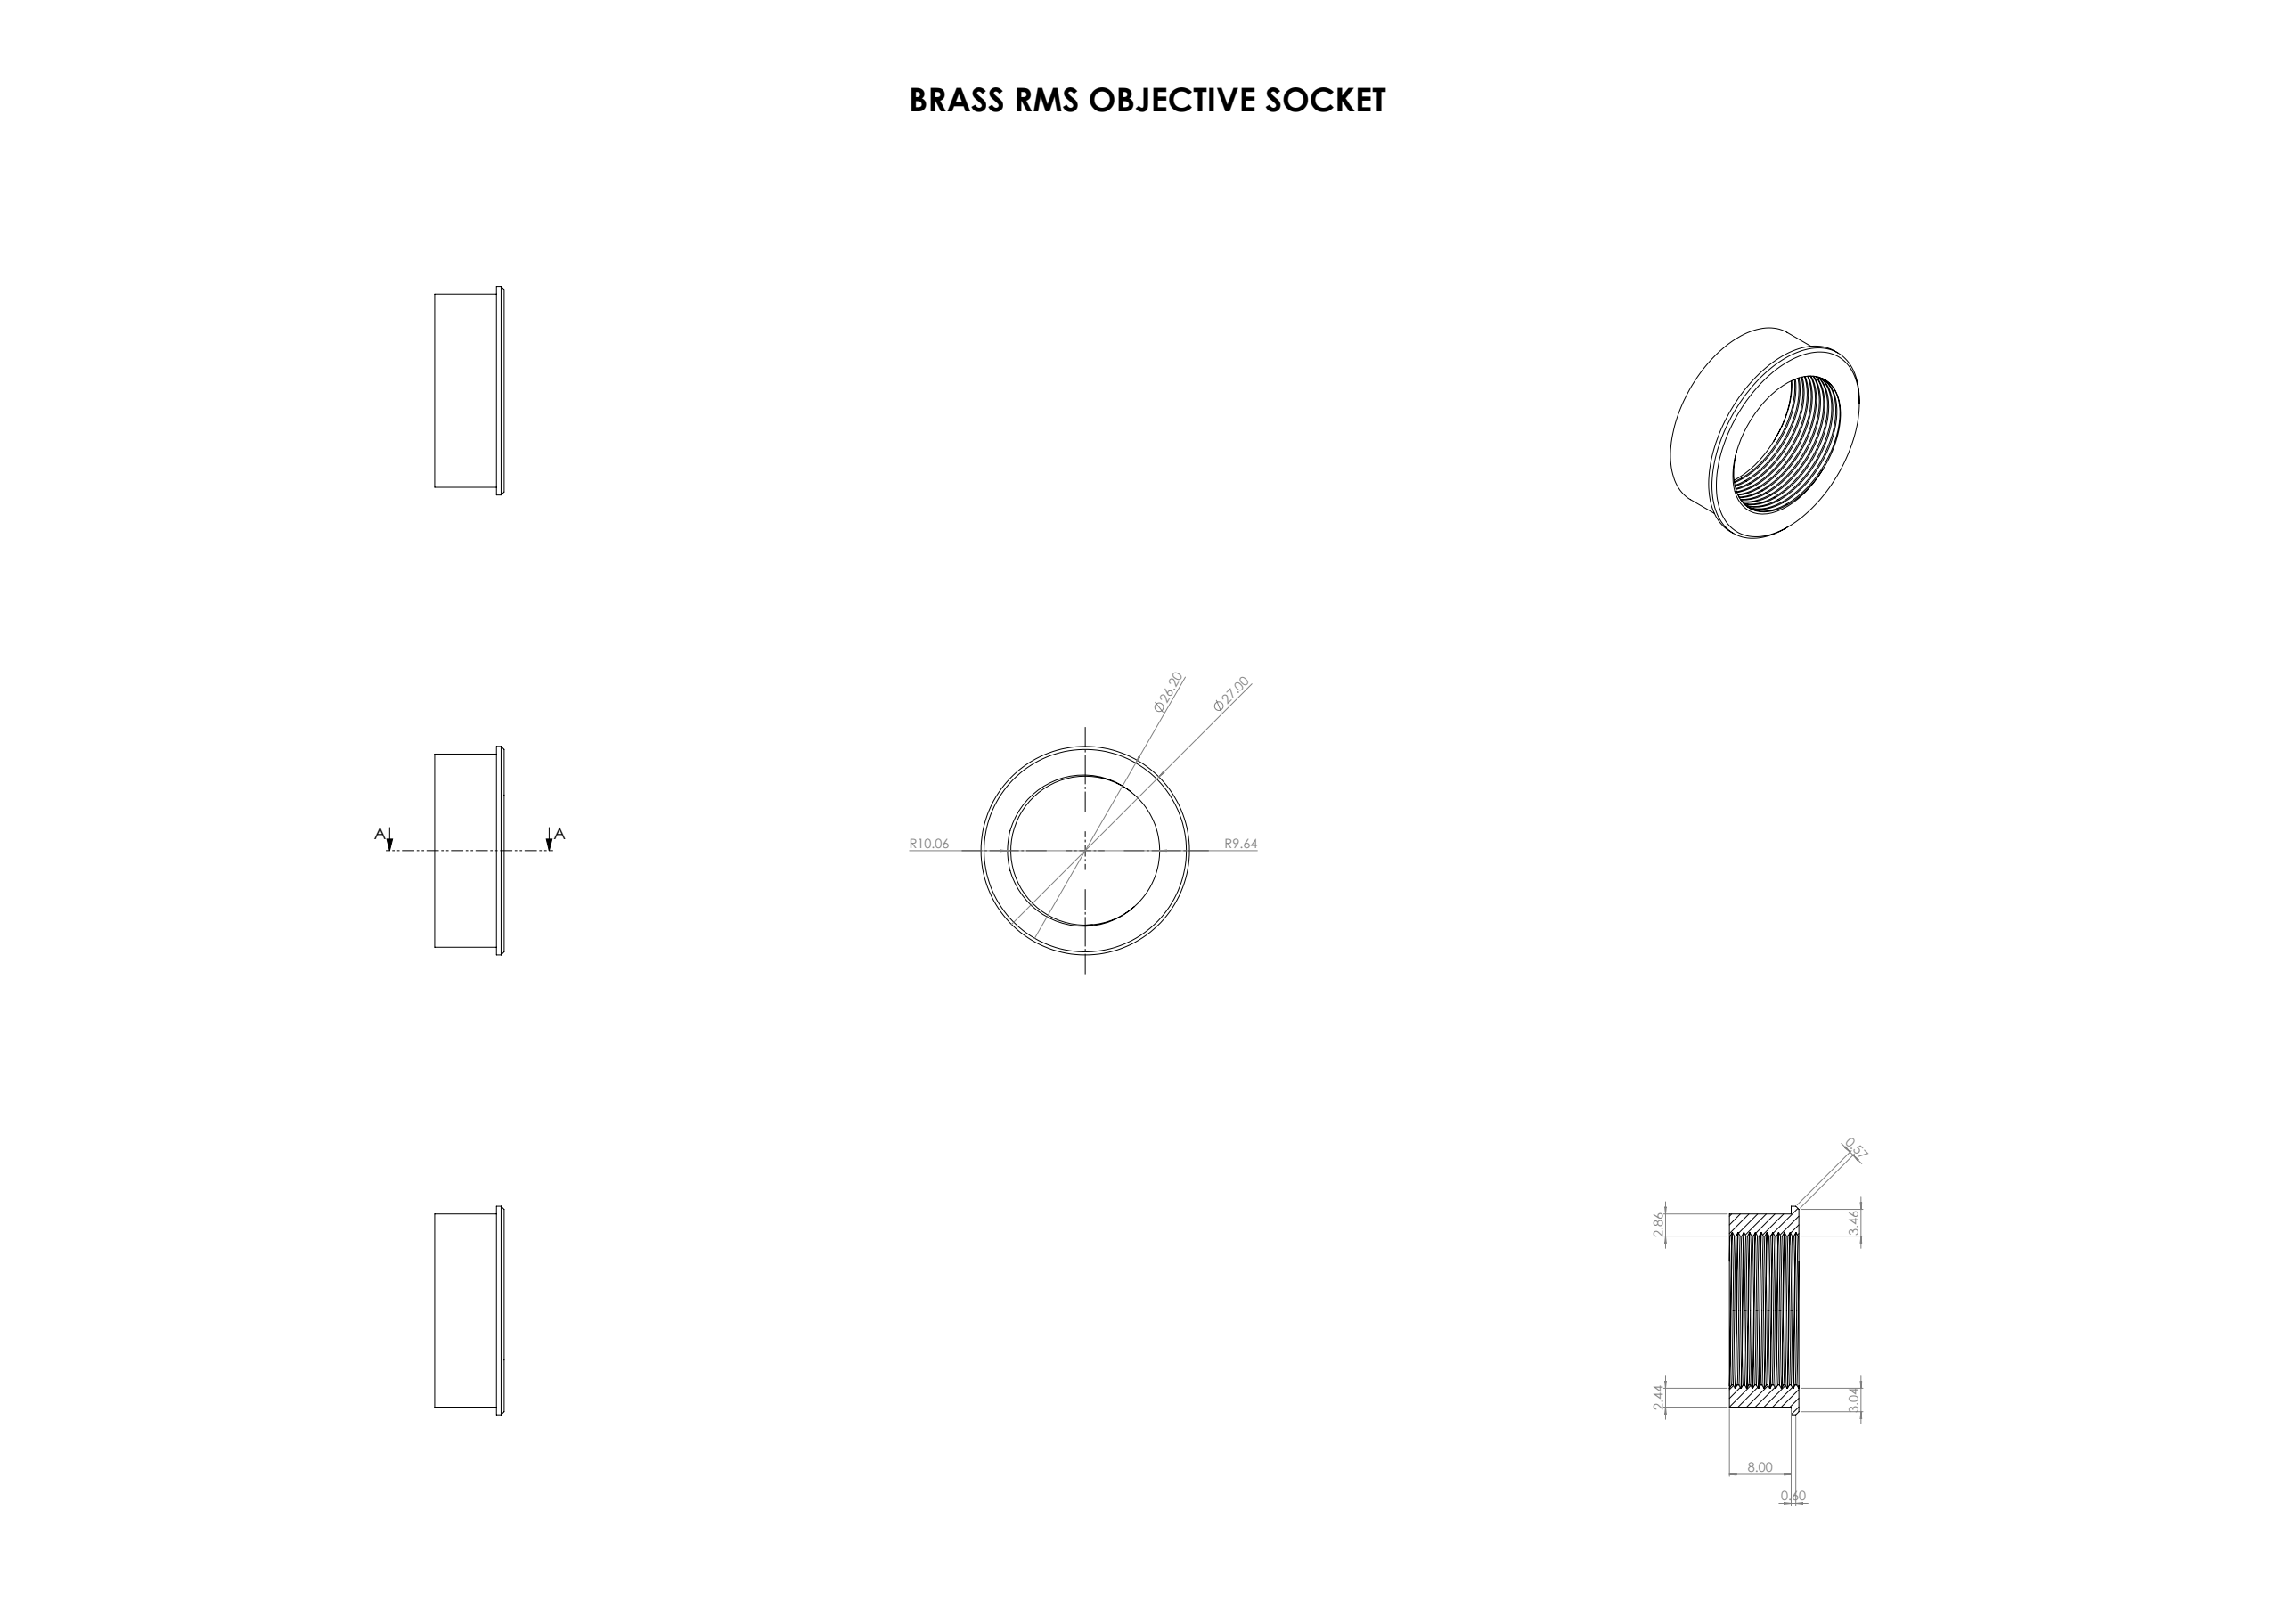
ISO-10303-21;
HEADER;
/* Generated by software containing ST-Developer
 * from STEP Tools, Inc. (www.steptools.com) 
 */

FILE_DESCRIPTION(
/* description */ (''),
/* implementation_level */ '2;1');

FILE_NAME(
/* name */ '03_Brass_RMS_Objective_Socket.step',
/* time_stamp */ '2026-10-21T02:03:06-07:00',
/* author */ (''),
/* organization */ (''),
/* preprocessor_version */ 'ST-DEVELOPER v20.2',
/* originating_system */ 'Autodesk Translation Framework v15.15.0.0',
/* authorisation */ '');

FILE_SCHEMA (('AUTOMOTIVE_DESIGN { 1 0 10303 214 3 1 1 }'));
ENDSEC;

DATA;
#10=MECHANICAL_DESIGN_GEOMETRIC_PRESENTATION_REPRESENTATION('',(#117),#38528);
#76=B_SPLINE_SURFACE_WITH_KNOTS('',3,3,((#30041,#30042,#30043,#30044,#30045,
#30046,#30047,#30048,#30049,#30050,#30051,#30052,#30053,#30054,#30055,#30056,
#30057,#30058,#30059,#30060,#30061,#30062,#30063,#30064,#30065,#30066,#30067,
#30068,#30069,#30070,#30071,#30072,#30073,#30074,#30075,#30076,#30077,#30078,
#30079,#30080,#30081,#30082,#30083,#30084,#30085,#30086,#30087,#30088,#30089,
#30090,#30091,#30092,#30093,#30094,#30095,#30096,#30097,#30098,#30099,#30100,
#30101,#30102,#30103,#30104,#30105,#30106,#30107,#30108,#30109,#30110,#30111,
#30112,#30113,#30114,#30115,#30116,#30117,#30118,#30119,#30120,#30121,#30122,
#30123,#30124,#30125,#30126,#30127,#30128,#30129,#30130,#30131,#30132,#30133,
#30134,#30135,#30136,#30137,#30138,#30139,#30140,#30141,#30142,#30143,#30144,
#30145,#30146,#30147,#30148,#30149,#30150,#30151,#30152,#30153,#30154,#30155,
#30156,#30157,#30158,#30159,#30160,#30161,#30162,#30163,#30164,#30165,#30166,
#30167,#30168,#30169,#30170,#30171,#30172,#30173,#30174,#30175,#30176,#30177,
#30178,#30179,#30180,#30181,#30182,#30183,#30184,#30185,#30186,#30187,#30188,
#30189,#30190,#30191,#30192,#30193,#30194,#30195,#30196,#30197,#30198,#30199),
(#30200,#30201,#30202,#30203,#30204,#30205,#30206,#30207,#30208,#30209,
#30210,#30211,#30212,#30213,#30214,#30215,#30216,#30217,#30218,#30219,#30220,
#30221,#30222,#30223,#30224,#30225,#30226,#30227,#30228,#30229,#30230,#30231,
#30232,#30233,#30234,#30235,#30236,#30237,#30238,#30239,#30240,#30241,#30242,
#30243,#30244,#30245,#30246,#30247,#30248,#30249,#30250,#30251,#30252,#30253,
#30254,#30255,#30256,#30257,#30258,#30259,#30260,#30261,#30262,#30263,#30264,
#30265,#30266,#30267,#30268,#30269,#30270,#30271,#30272,#30273,#30274,#30275,
#30276,#30277,#30278,#30279,#30280,#30281,#30282,#30283,#30284,#30285,#30286,
#30287,#30288,#30289,#30290,#30291,#30292,#30293,#30294,#30295,#30296,#30297,
#30298,#30299,#30300,#30301,#30302,#30303,#30304,#30305,#30306,#30307,#30308,
#30309,#30310,#30311,#30312,#30313,#30314,#30315,#30316,#30317,#30318,#30319,
#30320,#30321,#30322,#30323,#30324,#30325,#30326,#30327,#30328,#30329,#30330,
#30331,#30332,#30333,#30334,#30335,#30336,#30337,#30338,#30339,#30340,#30341,
#30342,#30343,#30344,#30345,#30346,#30347,#30348,#30349,#30350,#30351,#30352,
#30353,#30354,#30355,#30356,#30357,#30358),(#30359,#30360,#30361,#30362,
#30363,#30364,#30365,#30366,#30367,#30368,#30369,#30370,#30371,#30372,#30373,
#30374,#30375,#30376,#30377,#30378,#30379,#30380,#30381,#30382,#30383,#30384,
#30385,#30386,#30387,#30388,#30389,#30390,#30391,#30392,#30393,#30394,#30395,
#30396,#30397,#30398,#30399,#30400,#30401,#30402,#30403,#30404,#30405,#30406,
#30407,#30408,#30409,#30410,#30411,#30412,#30413,#30414,#30415,#30416,#30417,
#30418,#30419,#30420,#30421,#30422,#30423,#30424,#30425,#30426,#30427,#30428,
#30429,#30430,#30431,#30432,#30433,#30434,#30435,#30436,#30437,#30438,#30439,
#30440,#30441,#30442,#30443,#30444,#30445,#30446,#30447,#30448,#30449,#30450,
#30451,#30452,#30453,#30454,#30455,#30456,#30457,#30458,#30459,#30460,#30461,
#30462,#30463,#30464,#30465,#30466,#30467,#30468,#30469,#30470,#30471,#30472,
#30473,#30474,#30475,#30476,#30477,#30478,#30479,#30480,#30481,#30482,#30483,
#30484,#30485,#30486,#30487,#30488,#30489,#30490,#30491,#30492,#30493,#30494,
#30495,#30496,#30497,#30498,#30499,#30500,#30501,#30502,#30503,#30504,#30505,
#30506,#30507,#30508,#30509,#30510,#30511,#30512,#30513,#30514,#30515,#30516,
#30517),(#30518,#30519,#30520,#30521,#30522,#30523,#30524,#30525,#30526,
#30527,#30528,#30529,#30530,#30531,#30532,#30533,#30534,#30535,#30536,#30537,
#30538,#30539,#30540,#30541,#30542,#30543,#30544,#30545,#30546,#30547,#30548,
#30549,#30550,#30551,#30552,#30553,#30554,#30555,#30556,#30557,#30558,#30559,
#30560,#30561,#30562,#30563,#30564,#30565,#30566,#30567,#30568,#30569,#30570,
#30571,#30572,#30573,#30574,#30575,#30576,#30577,#30578,#30579,#30580,#30581,
#30582,#30583,#30584,#30585,#30586,#30587,#30588,#30589,#30590,#30591,#30592,
#30593,#30594,#30595,#30596,#30597,#30598,#30599,#30600,#30601,#30602,#30603,
#30604,#30605,#30606,#30607,#30608,#30609,#30610,#30611,#30612,#30613,#30614,
#30615,#30616,#30617,#30618,#30619,#30620,#30621,#30622,#30623,#30624,#30625,
#30626,#30627,#30628,#30629,#30630,#30631,#30632,#30633,#30634,#30635,#30636,
#30637,#30638,#30639,#30640,#30641,#30642,#30643,#30644,#30645,#30646,#30647,
#30648,#30649,#30650,#30651,#30652,#30653,#30654,#30655,#30656,#30657,#30658,
#30659,#30660,#30661,#30662,#30663,#30664,#30665,#30666,#30667,#30668,#30669,
#30670,#30671,#30672,#30673,#30674,#30675,#30676)),.UNSPECIFIED.,.F.,.F.,
 .F.,(4,4),(4,1,1,1,1,1,1,1,1,1,1,1,1,1,1,1,1,1,1,1,1,1,1,1,1,1,1,1,1,1,
1,1,1,1,1,1,1,1,1,1,1,1,1,1,1,1,1,1,1,1,1,1,1,1,1,1,1,1,1,1,1,1,1,1,1,1,
1,1,1,1,1,1,1,1,1,1,1,1,1,1,1,1,1,1,1,1,1,1,1,1,1,1,1,1,1,1,1,1,1,1,1,1,
1,1,1,1,1,1,1,1,1,1,1,1,1,1,1,1,1,1,1,1,1,1,1,1,1,1,1,1,1,1,1,1,1,1,1,1,
1,1,1,1,1,1,1,1,1,1,1,1,1,1,1,1,1,1,4),(0.,0.0485551576388473),(11.8415763884111,
12.3379359869576,12.8342955855041,13.3306551840506,13.827014782597,14.3233743811435,
14.81973397969,15.3160935782364,15.8124531767829,16.3088127753294,16.8051723738759,
17.3015319724223,17.7978915709688,18.2942511695153,18.7906107680618,19.2869703666082,
19.7833299651547,20.2796895637012,20.7760491622476,21.2724087607941,21.7687683593406,
22.2651279578871,22.7614875564335,23.25784715498,23.7542067535265,24.2505663520729,
24.7469259506194,25.2432855491659,25.7396451477124,26.2360047462588,26.7323643448053,
27.2287239433518,27.7250835418983,28.2214431404447,28.7178027389912,29.2141623375377,
29.7105219360841,30.2068815346306,30.7032411331771,31.1996007317236,31.69596033027,
32.1923199288165,32.688679527363,33.1850391259094,33.6813987244559,34.1777583230024,
34.6741179215489,35.1704775200953,35.6668371186418,36.1631967171883,36.6595563157347,
37.1559159142812,37.6522755128277,38.1486351113742,38.6449947099206,39.1413543084671,
39.6377139070136,40.1340735055601,40.6304331041065,41.126792702653,41.6231523011995,
42.1195118997459,42.6158714982924,43.1122310968389,43.6085906953854,44.1049502939318,
44.6013098924783,45.0976694910248,45.5940290895712,46.0903886881177,46.5867482866642,
47.0831078852107,47.5794674837571,48.0758270823036,48.5721866808501,49.0685462793965,
49.564905877943,50.0612654764895,50.557625075036,51.0539846735824,51.5503442721289,
52.0467038706754,52.5430634692219,53.0394230677683,53.5357826663148,54.0321422648613,
54.5285018634077,55.0248614619542,55.5212210605007,56.0175806590472,56.5139402575936,
57.0102998561401,57.5066594546866,58.003019053233,58.4993786517795,58.995738250326,
59.4920978488725,59.9884574474189,60.4848170459654,60.9811766445119,61.4775362430584,
61.9738958416048,62.4702554401513,62.9666150386978,63.4629746372442,63.9593342357907,
64.4556938343372,64.9520534328837,65.4484130314301,65.9447726299766,66.4411322285231,
66.9374918270696,67.433851425616,67.9302110241625,68.426570622709,68.9229302212554,
69.4192898198019,69.9156494183484,70.4120090168948,70.9083686154413,71.4047282139878,
71.9010878125343,72.3974474110807,72.8938070096272,73.3901666081737,73.8865262067201,
74.3828858052666,74.8792454038131,75.3756050023596,75.871964600906,76.3683241994525,
76.864683797999,77.3610433965455,77.8574029950919,78.3537625936384,78.8501221921849,
79.3464817907313,79.8428413892778,80.3392009878243,80.8355605863708,81.3319201849172,
81.8282797834637,82.3246393820102,82.8209989805567,83.3173585791031,83.8137181776496,
84.3100777761961,84.8064373747425,85.302796973289,85.7991565718355,86.295516170382,
86.7918757689284,87.2882353674749,87.7845949660214,88.2809545645678,88.7773141631143,
89.2736737616608),.UNSPECIFIED.);
#77=B_SPLINE_SURFACE_WITH_KNOTS('',3,3,((#30959,#30960,#30961,#30962,#30963,
#30964,#30965,#30966,#30967,#30968,#30969,#30970,#30971,#30972,#30973,#30974,
#30975,#30976,#30977,#30978,#30979,#30980,#30981,#30982,#30983,#30984,#30985,
#30986,#30987,#30988,#30989,#30990,#30991,#30992,#30993,#30994,#30995,#30996,
#30997,#30998,#30999,#31000,#31001,#31002,#31003,#31004,#31005,#31006,#31007,
#31008,#31009,#31010,#31011,#31012,#31013,#31014,#31015,#31016,#31017,#31018,
#31019,#31020,#31021,#31022,#31023,#31024,#31025,#31026,#31027,#31028,#31029,
#31030,#31031,#31032,#31033,#31034,#31035,#31036,#31037,#31038,#31039,#31040,
#31041,#31042,#31043,#31044,#31045,#31046,#31047,#31048,#31049,#31050,#31051,
#31052,#31053,#31054,#31055,#31056,#31057,#31058,#31059,#31060,#31061,#31062,
#31063,#31064,#31065,#31066,#31067,#31068,#31069,#31070,#31071,#31072,#31073,
#31074,#31075,#31076,#31077,#31078,#31079,#31080,#31081,#31082,#31083,#31084,
#31085,#31086,#31087,#31088,#31089,#31090,#31091,#31092,#31093,#31094,#31095,
#31096,#31097,#31098,#31099,#31100,#31101,#31102,#31103,#31104,#31105,#31106,
#31107,#31108,#31109,#31110,#31111,#31112,#31113,#31114,#31115,#31116,#31117),
(#31118,#31119,#31120,#31121,#31122,#31123,#31124,#31125,#31126,#31127,
#31128,#31129,#31130,#31131,#31132,#31133,#31134,#31135,#31136,#31137,#31138,
#31139,#31140,#31141,#31142,#31143,#31144,#31145,#31146,#31147,#31148,#31149,
#31150,#31151,#31152,#31153,#31154,#31155,#31156,#31157,#31158,#31159,#31160,
#31161,#31162,#31163,#31164,#31165,#31166,#31167,#31168,#31169,#31170,#31171,
#31172,#31173,#31174,#31175,#31176,#31177,#31178,#31179,#31180,#31181,#31182,
#31183,#31184,#31185,#31186,#31187,#31188,#31189,#31190,#31191,#31192,#31193,
#31194,#31195,#31196,#31197,#31198,#31199,#31200,#31201,#31202,#31203,#31204,
#31205,#31206,#31207,#31208,#31209,#31210,#31211,#31212,#31213,#31214,#31215,
#31216,#31217,#31218,#31219,#31220,#31221,#31222,#31223,#31224,#31225,#31226,
#31227,#31228,#31229,#31230,#31231,#31232,#31233,#31234,#31235,#31236,#31237,
#31238,#31239,#31240,#31241,#31242,#31243,#31244,#31245,#31246,#31247,#31248,
#31249,#31250,#31251,#31252,#31253,#31254,#31255,#31256,#31257,#31258,#31259,
#31260,#31261,#31262,#31263,#31264,#31265,#31266,#31267,#31268,#31269,#31270,
#31271,#31272,#31273,#31274,#31275,#31276),(#31277,#31278,#31279,#31280,
#31281,#31282,#31283,#31284,#31285,#31286,#31287,#31288,#31289,#31290,#31291,
#31292,#31293,#31294,#31295,#31296,#31297,#31298,#31299,#31300,#31301,#31302,
#31303,#31304,#31305,#31306,#31307,#31308,#31309,#31310,#31311,#31312,#31313,
#31314,#31315,#31316,#31317,#31318,#31319,#31320,#31321,#31322,#31323,#31324,
#31325,#31326,#31327,#31328,#31329,#31330,#31331,#31332,#31333,#31334,#31335,
#31336,#31337,#31338,#31339,#31340,#31341,#31342,#31343,#31344,#31345,#31346,
#31347,#31348,#31349,#31350,#31351,#31352,#31353,#31354,#31355,#31356,#31357,
#31358,#31359,#31360,#31361,#31362,#31363,#31364,#31365,#31366,#31367,#31368,
#31369,#31370,#31371,#31372,#31373,#31374,#31375,#31376,#31377,#31378,#31379,
#31380,#31381,#31382,#31383,#31384,#31385,#31386,#31387,#31388,#31389,#31390,
#31391,#31392,#31393,#31394,#31395,#31396,#31397,#31398,#31399,#31400,#31401,
#31402,#31403,#31404,#31405,#31406,#31407,#31408,#31409,#31410,#31411,#31412,
#31413,#31414,#31415,#31416,#31417,#31418,#31419,#31420,#31421,#31422,#31423,
#31424,#31425,#31426,#31427,#31428,#31429,#31430,#31431,#31432,#31433,#31434,
#31435),(#31436,#31437,#31438,#31439,#31440,#31441,#31442,#31443,#31444,
#31445,#31446,#31447,#31448,#31449,#31450,#31451,#31452,#31453,#31454,#31455,
#31456,#31457,#31458,#31459,#31460,#31461,#31462,#31463,#31464,#31465,#31466,
#31467,#31468,#31469,#31470,#31471,#31472,#31473,#31474,#31475,#31476,#31477,
#31478,#31479,#31480,#31481,#31482,#31483,#31484,#31485,#31486,#31487,#31488,
#31489,#31490,#31491,#31492,#31493,#31494,#31495,#31496,#31497,#31498,#31499,
#31500,#31501,#31502,#31503,#31504,#31505,#31506,#31507,#31508,#31509,#31510,
#31511,#31512,#31513,#31514,#31515,#31516,#31517,#31518,#31519,#31520,#31521,
#31522,#31523,#31524,#31525,#31526,#31527,#31528,#31529,#31530,#31531,#31532,
#31533,#31534,#31535,#31536,#31537,#31538,#31539,#31540,#31541,#31542,#31543,
#31544,#31545,#31546,#31547,#31548,#31549,#31550,#31551,#31552,#31553,#31554,
#31555,#31556,#31557,#31558,#31559,#31560,#31561,#31562,#31563,#31564,#31565,
#31566,#31567,#31568,#31569,#31570,#31571,#31572,#31573,#31574,#31575,#31576,
#31577,#31578,#31579,#31580,#31581,#31582,#31583,#31584,#31585,#31586,#31587,
#31588,#31589,#31590,#31591,#31592,#31593,#31594)),.UNSPECIFIED.,.F.,.F.,
 .F.,(4,4),(4,1,1,1,1,1,1,1,1,1,1,1,1,1,1,1,1,1,1,1,1,1,1,1,1,1,1,1,1,1,
1,1,1,1,1,1,1,1,1,1,1,1,1,1,1,1,1,1,1,1,1,1,1,1,1,1,1,1,1,1,1,1,1,1,1,1,
1,1,1,1,1,1,1,1,1,1,1,1,1,1,1,1,1,1,1,1,1,1,1,1,1,1,1,1,1,1,1,1,1,1,1,1,
1,1,1,1,1,1,1,1,1,1,1,1,1,1,1,1,1,1,1,1,1,1,1,1,1,1,1,1,1,1,1,1,1,1,1,1,
1,1,1,1,1,1,1,1,1,1,1,1,1,1,1,1,1,1,4),(0.,0.0485551576388473),(14.3988838068023,
14.8952434053488,15.3916030038952,15.8879626024417,16.3843222009882,16.8806817995346,
17.3770413980811,17.8734009966276,18.3697605951741,18.8661201937205,19.362479792267,
19.8588393908135,20.3551989893599,20.8515585879064,21.3479181864529,21.8442777849994,
22.3406373835458,22.8369969820923,23.3333565806388,23.8297161791853,24.3260757777317,
24.8224353762782,25.3187949748247,25.8151545733711,26.3115141719176,26.8078737704641,
27.3042333690106,27.800592967557,28.2969525661035,28.79331216465,29.2896717631964,
29.7860313617429,30.2823909602894,30.7787505588359,31.2751101573823,31.7714697559288,
32.2678293544753,32.7641889530218,33.2605485515682,33.7569081501147,34.2532677486612,
34.7496273472076,35.2459869457541,35.7423465443006,36.2387061428471,36.7350657413935,
37.23142533994,37.7277849384865,38.2241445370329,38.7205041355794,39.2168637341259,
39.7132233326724,40.2095829312188,40.7059425297653,41.2023021283118,41.6986617268582,
42.1950213254047,42.6913809239512,43.1877405224977,43.6841001210441,44.1804597195906,
44.6768193181371,45.1731789166836,45.66953851523,46.1658981137765,46.662257712323,
47.1586173108694,47.6549769094159,48.1513365079624,48.6476961065089,49.1440557050553,
49.6404153036018,50.1367749021483,50.6331345006947,51.1294940992412,51.6258536977877,
52.1222132963342,52.6185728948806,53.1149324934271,53.6112920919736,54.1076516905201,
54.6040112890665,55.100370887613,55.5967304861595,56.0930900847059,56.5894496832524,
57.0858092817989,57.5821688803454,58.0785284788918,58.5748880774383,59.0712476759848,
59.5676072745312,60.0639668730777,60.5603264716242,61.0566860701707,61.5530456687171,
62.0494052672636,62.5457648658101,63.0421244643565,63.538484062903,64.0348436614495,
64.531203259996,65.0275628585424,65.5239224570889,66.0202820556354,66.5166416541819,
67.0130012527283,67.5093608512748,68.0057204498213,68.5020800483677,68.9984396469142,
69.4947992454607,69.9911588440072,70.4875184425536,70.9838780411001,71.4802376396466,
71.9765972381931,72.4729568367395,72.969316435286,73.4656760338325,73.9620356323789,
74.4583952309254,74.9547548294719,75.4511144280183,75.9474740265648,76.4438336251113,
76.9401932236578,77.4365528222042,77.9329124207507,78.4292720192972,78.9256316178437,
79.4219912163901,79.9183508149366,80.4147104134831,80.9110700120296,81.407429610576,
81.9037892091225,82.400148807669,82.8965084062154,83.3928680047619,83.8892276033084,
84.3855872018549,84.8819468004013,85.3783063989478,85.8746659974943,86.3710255960407,
86.8673851945872,87.3637447931337,87.8601043916802,88.3564639902266,88.8528235887731,
89.3491831873196,89.845542785866,90.3419023844125,90.838261982959,91.3346215815055,
91.8309811800519),.UNSPECIFIED.);
#93=SHAPE_REPRESENTATION_RELATIONSHIP('SRR','None',#38578,#105);
#105=ADVANCED_BREP_SHAPE_REPRESENTATION('',(#129),#38518);
#117=STYLED_ITEM('',(#38692),#129);
#129=MANIFOLD_SOLID_BREP('Body1',#17074);
#334=CYLINDRICAL_SURFACE('',#18600,9.64155);
#335=CYLINDRICAL_SURFACE('',#18602,9.64155);
#336=CYLINDRICAL_SURFACE('',#18603,9.64155);
#337=CYLINDRICAL_SURFACE('',#18604,9.64155);
#338=CYLINDRICAL_SURFACE('',#18605,9.64155);
#339=CYLINDRICAL_SURFACE('',#18606,9.64155);
#340=CYLINDRICAL_SURFACE('',#18607,9.64155);
#341=CYLINDRICAL_SURFACE('',#18608,9.64155);
#342=CYLINDRICAL_SURFACE('',#18609,9.64155);
#343=CYLINDRICAL_SURFACE('',#18610,9.64155);
#344=CYLINDRICAL_SURFACE('',#18611,9.64155);
#345=CYLINDRICAL_SURFACE('',#18612,9.64155);
#346=CYLINDRICAL_SURFACE('',#18614,10.06205);
#347=CYLINDRICAL_SURFACE('',#18616,10.06205);
#348=CYLINDRICAL_SURFACE('',#18617,10.06205);
#349=CYLINDRICAL_SURFACE('',#18618,10.06205);
#350=CYLINDRICAL_SURFACE('',#18619,10.06205);
#351=CYLINDRICAL_SURFACE('',#18620,10.06205);
#352=CYLINDRICAL_SURFACE('',#18621,10.06205);
#353=CYLINDRICAL_SURFACE('',#18622,10.06205);
#354=CYLINDRICAL_SURFACE('',#18623,10.06205);
#355=CYLINDRICAL_SURFACE('',#18624,10.06205);
#356=CYLINDRICAL_SURFACE('',#18625,10.06205);
#357=CYLINDRICAL_SURFACE('',#18626,10.06205);
#358=CYLINDRICAL_SURFACE('',#18628,10.06205);
#359=CYLINDRICAL_SURFACE('',#18631,9.64155);
#360=CYLINDRICAL_SURFACE('',#18632,12.5);
#361=CYLINDRICAL_SURFACE('',#18636,13.5);
#631=B_SPLINE_CURVE_WITH_KNOTS('',3,(#28607,#28608,#28609,#28610,#28611,
#28612,#28613,#28614,#28615,#28616,#28617,#28618,#28619,#28620,#28621,#28622,
#28623,#28624,#28625,#28626,#28627,#28628,#28629,#28630,#28631),
 .UNSPECIFIED.,.F.,.F.,(4,3,3,3,3,3,3,3,4),(-3.86638687953777,-3.47451718982531,
-2.97815759127883,-2.48179799273236,-1.98543839418589,-1.48907879563941,
-0.992719197092944,-0.496359598546473,0.),.UNSPECIFIED.);
#632=B_SPLINE_CURVE_WITH_KNOTS('',3,(#28634,#28635,#28636,#28637,#28638,
#28639,#28640,#28641,#28642,#28643,#28644,#28645,#28646,#28647,#28648,#28649,
#28650,#28651,#28652,#28653,#28654,#28655,#28656,#28657,#28658,#28659,#28660,
#28661,#28662,#28663,#28664,#28665,#28666,#28667,#28668,#28669,#28670),
 .UNSPECIFIED.,.F.,.F.,(4,3,3,3,3,3,3,3,3,3,3,3,4),(2.03387368709462,2.48179799273236,
2.97815759127883,3.4745171898253,3.97087678837177,4.46723638691825,4.96359598546472,
5.4599555840112,5.95631518255767,6.45267478110414,6.94903437965062,7.44539397819709,
7.59226476832617),.UNSPECIFIED.);
#633=B_SPLINE_CURVE_WITH_KNOTS('',3,(#28675,#28676,#28677,#28678,#28679,
#28680,#28681,#28682,#28683,#28684,#28685,#28686,#28687,#28688,#28689,#28690,
#28691,#28692,#28693,#28694,#28695,#28696,#28697,#28698,#28699,#28700,#28701,
#28702,#28703,#28704,#28705,#28706,#28707,#28708,#28709,#28710,#28711,#28712,
#28713,#28714,#28715,#28716,#28717),.UNSPECIFIED.,.F.,.F.,(4,3,3,3,3,3,
3,3,3,3,3,3,3,3,4),(-10.1495721867174,-9.92719197092945,-9.43083237238297,
-8.9344727738365,-8.43811317529003,-7.94175357674355,-7.44539397819708,
-6.94903437965061,-6.45267478110414,-5.95631518255767,-5.45995558401119,
-4.96359598546472,-4.46723638691825,-3.97087678837178,-3.86638687953777),
 .UNSPECIFIED.);
#634=B_SPLINE_CURVE_WITH_KNOTS('',3,(#28718,#28719,#28720,#28721,#28722,
#28723,#28724,#28725,#28726,#28727,#28728,#28729,#28730,#28731,#28732,#28733,
#28734,#28735,#28736,#28737,#28738,#28739,#28740,#28741,#28742,#28743,#28744,
#28745,#28746,#28747,#28748,#28749,#28750,#28751,#28752,#28753,#28754,#28755,
#28756,#28757),.UNSPECIFIED.,.F.,.F.,(4,3,3,3,3,3,3,3,3,3,3,3,3,4),(7.59226476832617,
7.94175357674356,8.43811317529003,8.93447277383651,9.43083237238297,9.92719197092945,
10.4235515694759,10.9199111680224,11.4162707665689,11.9126303651153,12.4089899636618,
12.9053495622083,13.4017091607548,13.8754500755058),.UNSPECIFIED.);
#635=B_SPLINE_CURVE_WITH_KNOTS('',3,(#28762,#28763,#28764,#28765,#28766,
#28767,#28768,#28769,#28770,#28771,#28772,#28773,#28774,#28775,#28776,#28777,
#28778,#28779,#28780,#28781,#28782,#28783,#28784,#28785,#28786,#28787,#28788,
#28789,#28790,#28791,#28792,#28793,#28794,#28795,#28796,#28797,#28798,#28799,
#28800,#28801,#28802,#28803,#28804),.UNSPECIFIED.,.F.,.F.,(4,3,3,3,3,3,
3,3,3,3,3,3,3,3,4),(-16.432757493897,-16.3798667520336,-15.8835071534871,
-15.3871475549406,-14.8907879563942,-14.3944283578477,-13.8980687593012,
-13.4017091607547,-12.9053495622083,-12.4089899636618,-11.9126303651153,
-11.4162707665689,-10.9199111680224,-10.4235515694759,-10.1495721867174),
 .UNSPECIFIED.);
#636=B_SPLINE_CURVE_WITH_KNOTS('',3,(#28805,#28806,#28807,#28808,#28809,
#28810,#28811,#28812,#28813,#28814,#28815,#28816,#28817,#28818,#28819,#28820,
#28821,#28822,#28823,#28824,#28825,#28826,#28827,#28828,#28829,#28830,#28831,
#28832,#28833,#28834,#28835,#28836,#28837,#28838,#28839,#28840,#28841,#28842,
#28843,#28844,#28845,#28846,#28847),.UNSPECIFIED.,.F.,.F.,(4,3,3,3,3,3,
3,3,3,3,3,3,3,3,4),(13.8754500755058,13.8980687593012,14.3944283578477,
14.8907879563942,15.3871475549406,15.8835071534871,16.3798667520336,16.87622635058,
17.3725859491265,17.868945547673,18.3653051462195,18.8616647447659,19.3580243433124,
19.8543839418589,20.1586353826853),.UNSPECIFIED.);
#637=B_SPLINE_CURVE_WITH_KNOTS('',3,(#28852,#28853,#28854,#28855,#28856,
#28857,#28858,#28859,#28860,#28861,#28862,#28863,#28864,#28865,#28866,#28867,
#28868,#28869,#28870,#28871,#28872,#28873,#28874,#28875,#28876,#28877,#28878,
#28879,#28880,#28881,#28882,#28883,#28884,#28885,#28886,#28887,#28888,#28889,
#28890,#28891),.UNSPECIFIED.,.F.,.F.,(4,3,3,3,3,3,3,3,3,3,3,3,3,4),(-22.7159428010765,
-22.3361819345912,-21.8398223360448,-21.3434627374983,-20.8471031389518,
-20.3507435404054,-19.8543839418589,-19.3580243433124,-18.8616647447659,
-18.3653051462195,-17.868945547673,-17.3725859491265,-16.8762263505801,
-16.432757493897),.UNSPECIFIED.);
#638=B_SPLINE_CURVE_WITH_KNOTS('',3,(#28892,#28893,#28894,#28895,#28896,
#28897,#28898,#28899,#28900,#28901,#28902,#28903,#28904,#28905,#28906,#28907,
#28908,#28909,#28910,#28911,#28912,#28913,#28914,#28915,#28916,#28917,#28918,
#28919,#28920,#28921,#28922,#28923,#28924,#28925,#28926,#28927,#28928,#28929,
#28930,#28931,#28932,#28933,#28934),.UNSPECIFIED.,.F.,.F.,(4,3,3,3,3,3,
3,3,3,3,3,3,3,3,4),(20.1586353826853,20.3507435404054,20.8471031389518,
21.3434627374983,21.8398223360448,22.3361819345912,22.8325415331377,23.3289011316842,
23.8252607302307,24.3216203287771,24.8179799273236,25.3143395258701,25.8106991244165,
26.307058722963,26.4418206898649),.UNSPECIFIED.);
#639=B_SPLINE_CURVE_WITH_KNOTS('',3,(#28939,#28940,#28941,#28942,#28943,
#28944,#28945,#28946,#28947,#28948,#28949,#28950,#28951,#28952,#28953,#28954,
#28955,#28956,#28957,#28958,#28959,#28960,#28961,#28962,#28963,#28964,#28965,
#28966,#28967,#28968,#28969,#28970,#28971,#28972,#28973,#28974,#28975,#28976,
#28977,#28978,#28979,#28980,#28981),.UNSPECIFIED.,.F.,.F.,(4,3,3,3,3,3,
3,3,3,3,3,3,3,3,4),(-28.9991281082561,-28.7888567156954,-28.2924971171489,
-27.7961375186024,-27.299777920056,-26.8034183215095,-26.307058722963,-25.8106991244165,
-25.3143395258701,-24.8179799273236,-24.3216203287771,-23.8252607302307,
-23.3289011316842,-22.8325415331377,-22.7159428010765),.UNSPECIFIED.);
#640=B_SPLINE_CURVE_WITH_KNOTS('',3,(#28982,#28983,#28984,#28985,#28986,
#28987,#28988,#28989,#28990,#28991,#28992,#28993,#28994,#28995,#28996,#28997,
#28998,#28999,#29000,#29001,#29002,#29003,#29004,#29005,#29006,#29007,#29008,
#29009,#29010,#29011,#29012,#29013,#29014,#29015,#29016,#29017,#29018,#29019,
#29020,#29021),.UNSPECIFIED.,.F.,.F.,(4,3,3,3,3,3,3,3,3,3,3,3,3,4),(26.4418206898649,
26.8034183215095,27.299777920056,27.7961375186024,28.2924971171489,28.7888567156954,
29.2852163142419,29.7815759127883,30.2779355113348,30.7742951098813,31.2706547084277,
31.7670143069742,32.2633739055207,32.7250059970445),.UNSPECIFIED.);
#641=B_SPLINE_CURVE_WITH_KNOTS('',3,(#29026,#29027,#29028,#29029,#29030,
#29031,#29032,#29033,#29034,#29035,#29036,#29037,#29038,#29039,#29040,#29041,
#29042,#29043,#29044,#29045,#29046,#29047,#29048,#29049,#29050,#29051,#29052,
#29053,#29054,#29055,#29056,#29057,#29058,#29059,#29060,#29061,#29062,#29063,
#29064,#29065,#29066,#29067,#29068),.UNSPECIFIED.,.F.,.F.,(4,3,3,3,3,3,
3,3,3,3,3,3,3,3,4),(-35.2823134154357,-35.2415314967995,-34.745171898253,
-34.2488122997066,-33.7524527011601,-33.2560931026136,-32.7597335040672,
-32.2633739055207,-31.7670143069742,-31.2706547084277,-30.7742951098813,
-30.2779355113348,-29.7815759127883,-29.2852163142419,-28.9991281082561),
 .UNSPECIFIED.);
#642=B_SPLINE_CURVE_WITH_KNOTS('',3,(#29069,#29070,#29071,#29072,#29073,
#29074,#29075,#29076,#29077,#29078,#29079,#29080,#29081,#29082,#29083,#29084,
#29085,#29086,#29087,#29088,#29089,#29090,#29091,#29092,#29093,#29094,#29095,
#29096,#29097,#29098,#29099,#29100,#29101,#29102,#29103,#29104,#29105,#29106,
#29107,#29108,#29109,#29110,#29111),.UNSPECIFIED.,.F.,.F.,(4,3,3,3,3,3,
3,3,3,3,3,3,3,3,4),(32.7250059970445,32.7597335040672,33.2560931026136,
33.7524527011601,34.2488122997066,34.7451718982531,35.2415314967995,35.737891095346,
36.2342506938925,36.7306102924389,37.2269698909854,37.7233294895319,38.2196890880783,
38.7160486866248,39.0081913042241),.UNSPECIFIED.);
#643=B_SPLINE_CURVE_WITH_KNOTS('',3,(#29116,#29117,#29118,#29119,#29120,
#29121,#29122,#29123,#29124,#29125,#29126,#29127,#29128,#29129,#29130,#29131,
#29132,#29133,#29134,#29135,#29136,#29137,#29138,#29139,#29140,#29141,#29142,
#29143,#29144,#29145,#29146,#29147,#29148,#29149,#29150,#29151,#29152,#29153,
#29154,#29155),.UNSPECIFIED.,.F.,.F.,(4,3,3,3,3,3,3,3,3,3,3,3,3,4),(-41.5654987226153,
-41.1978466793572,-40.7014870808107,-40.2051274822642,-39.7087678837178,
-39.2124082851713,-38.7160486866248,-38.2196890880784,-37.7233294895319,
-37.2269698909854,-36.7306102924389,-36.2342506938925,-35.737891095346,
-35.2823134154357),.UNSPECIFIED.);
#644=B_SPLINE_CURVE_WITH_KNOTS('',3,(#29156,#29157,#29158,#29159,#29160,
#29161,#29162,#29163,#29164,#29165,#29166,#29167,#29168,#29169,#29170,#29171,
#29172,#29173,#29174,#29175,#29176,#29177,#29178,#29179,#29180,#29181,#29182,
#29183,#29184,#29185,#29186,#29187,#29188,#29189,#29190,#29191,#29192,#29193,
#29194,#29195,#29196,#29197,#29198),.UNSPECIFIED.,.F.,.F.,(4,3,3,3,3,3,
3,3,3,3,3,3,3,3,4),(39.0081913042241,39.2124082851713,39.7087678837178,
40.2051274822642,40.7014870808107,41.1978466793572,41.6942062779036,42.1905658764501,
42.6869254749966,43.1832850735431,43.6796446720895,44.176004270636,44.6723638691825,
45.168723467729,45.2913766114037),.UNSPECIFIED.);
#645=B_SPLINE_CURVE_WITH_KNOTS('',3,(#29203,#29204,#29205,#29206,#29207,
#29208,#29209,#29210,#29211,#29212,#29213,#29214,#29215,#29216,#29217,#29218,
#29219,#29220,#29221,#29222,#29223,#29224,#29225,#29226,#29227,#29228,#29229,
#29230,#29231,#29232,#29233,#29234,#29235,#29236,#29237,#29238,#29239,#29240,
#29241,#29242,#29243,#29244,#29245),.UNSPECIFIED.,.F.,.F.,(4,3,3,3,3,3,
3,3,3,3,3,3,3,3,4),(-47.8486840297949,-47.6505214604613,-47.1541618619148,
-46.6578022633684,-46.1614426648219,-45.6650830662754,-45.168723467729,
-44.6723638691825,-44.176004270636,-43.6796446720895,-43.1832850735431,
-42.6869254749966,-42.1905658764501,-41.6942062779037,-41.5654987226153),
 .UNSPECIFIED.);
#646=B_SPLINE_CURVE_WITH_KNOTS('',3,(#29246,#29247,#29248,#29249,#29250,
#29251,#29252,#29253,#29254,#29255,#29256,#29257,#29258,#29259,#29260,#29261,
#29262,#29263,#29264,#29265,#29266,#29267,#29268,#29269,#29270,#29271,#29272,
#29273,#29274,#29275,#29276,#29277,#29278,#29279,#29280,#29281,#29282,#29283,
#29284,#29285),.UNSPECIFIED.,.F.,.F.,(4,3,3,3,3,3,3,3,3,3,3,3,3,4),(45.2913766114037,
45.6650830662754,46.1614426648219,46.6578022633684,47.1541618619148,47.6505214604613,
48.1468810590078,48.6432406575543,49.1396002561007,49.6359598546472,50.1323194531937,
50.6286790517402,51.1250386502866,51.5745619185833),.UNSPECIFIED.);
#647=B_SPLINE_CURVE_WITH_KNOTS('',3,(#29290,#29291,#29292,#29293,#29294,
#29295,#29296,#29297,#29298,#29299,#29300,#29301,#29302,#29303,#29304,#29305,
#29306,#29307,#29308,#29309,#29310,#29311,#29312,#29313,#29314,#29315,#29316,
#29317,#29318,#29319,#29320,#29321,#29322,#29323,#29324,#29325,#29326,#29327,
#29328,#29329,#29330,#29331,#29332),.UNSPECIFIED.,.F.,.F.,(4,3,3,3,3,3,
3,3,3,3,3,3,3,3,4),(-54.1318693369745,-54.1031962415655,-53.606836643019,
-53.1104770444725,-52.614117445926,-52.1177578473796,-51.6213982488331,
-51.1250386502866,-50.6286790517402,-50.1323194531937,-49.6359598546472,
-49.1396002561007,-48.6432406575543,-48.1468810590078,-47.8486840297949),
 .UNSPECIFIED.);
#648=B_SPLINE_CURVE_WITH_KNOTS('',3,(#29333,#29334,#29335,#29336,#29337,
#29338,#29339,#29340,#29341,#29342,#29343,#29344,#29345,#29346,#29347,#29348,
#29349,#29350,#29351,#29352,#29353,#29354,#29355,#29356,#29357,#29358,#29359,
#29360,#29361,#29362,#29363,#29364,#29365,#29366,#29367,#29368,#29369,#29370,
#29371,#29372,#29373,#29374,#29375),.UNSPECIFIED.,.F.,.F.,(4,3,3,3,3,3,
3,3,3,3,3,3,3,3,4),(51.5745619185833,51.6213982488331,52.1177578473796,
52.6141174459261,53.1104770444725,53.606836643019,54.1031962415655,54.5995558401119,
55.0959154386584,55.5922750372049,56.0886346357514,56.5849942342978,57.0813538328443,
57.5777134313908,57.8577472257629),.UNSPECIFIED.);
#649=B_SPLINE_CURVE_WITH_KNOTS('',3,(#29380,#29381,#29382,#29383,#29384,
#29385,#29386,#29387,#29388,#29389,#29390,#29391,#29392,#29393,#29394,#29395,
#29396,#29397,#29398,#29399,#29400,#29401,#29402,#29403,#29404,#29405,#29406,
#29407,#29408,#29409,#29410,#29411,#29412,#29413,#29414,#29415,#29416,#29417,
#29418,#29419),.UNSPECIFIED.,.F.,.F.,(4,3,3,3,3,3,3,3,3,3,3,3,3,4),(-60.4150546441541,
-60.0595114241231,-59.5631518255767,-59.0667922270302,-58.5704326284837,
-58.0740730299372,-57.5777134313908,-57.0813538328443,-56.5849942342978,
-56.0886346357513,-55.5922750372049,-55.0959154386584,-54.5995558401119,
-54.1318693369745),.UNSPECIFIED.);
#650=B_SPLINE_CURVE_WITH_KNOTS('',3,(#29420,#29421,#29422,#29423,#29424,
#29425,#29426,#29427,#29428,#29429,#29430,#29431,#29432,#29433,#29434,#29435,
#29436,#29437,#29438,#29439,#29440,#29441,#29442,#29443,#29444,#29445,#29446,
#29447,#29448,#29449,#29450,#29451,#29452,#29453,#29454,#29455,#29456,#29457,
#29458,#29459,#29460,#29461,#29462),.UNSPECIFIED.,.F.,.F.,(4,3,3,3,3,3,
3,3,3,3,3,3,3,3,4),(57.8577472257629,58.0740730299372,58.5704326284837,
59.0667922270302,59.5631518255767,60.0595114241231,60.5558710226696,61.0522306212161,
61.5485902197625,62.044949818309,62.5413094168555,63.037669015402,63.5340286139484,
64.0303882124949,64.1409325329425),.UNSPECIFIED.);
#651=B_SPLINE_CURVE_WITH_KNOTS('',3,(#29467,#29468,#29469,#29470,#29471,
#29472,#29473,#29474,#29475,#29476,#29477,#29478,#29479,#29480,#29481,#29482,
#29483,#29484,#29485,#29486,#29487,#29488,#29489,#29490,#29491,#29492,#29493,
#29494,#29495,#29496,#29497,#29498,#29499,#29500,#29501,#29502,#29503,#29504,
#29505,#29506,#29507,#29508,#29509),.UNSPECIFIED.,.F.,.F.,(4,3,3,3,3,3,
3,3,3,3,3,3,3,3,4),(-66.6982399513337,-66.5121862052273,-66.0158266066808,
-65.5194670081343,-65.0231074095879,-64.5267478110414,-64.0303882124949,
-63.5340286139484,-63.037669015402,-62.5413094168555,-62.044949818309,-61.5485902197625,
-61.0522306212161,-60.5558710226696,-60.4150546441541),.UNSPECIFIED.);
#652=B_SPLINE_CURVE_WITH_KNOTS('',3,(#29510,#29511,#29512,#29513,#29514,
#29515,#29516,#29517,#29518,#29519,#29520,#29521,#29522,#29523,#29524,#29525,
#29526,#29527,#29528,#29529,#29530,#29531,#29532,#29533,#29534,#29535,#29536,
#29537,#29538,#29539,#29540,#29541,#29542,#29543,#29544,#29545,#29546,#29547,
#29548,#29549),.UNSPECIFIED.,.F.,.F.,(4,3,3,3,3,3,3,3,3,3,3,3,3,4),(64.1409325329425,
64.5267478110414,65.0231074095878,65.5194670081343,66.0158266066808,66.5121862052273,
67.0085458037737,67.5049054023202,68.0012650008667,68.4976245994131,68.9939841979596,
69.4903437965061,69.9867033950526,70.4241178401221),.UNSPECIFIED.);
#653=B_SPLINE_CURVE_WITH_KNOTS('',3,(#29555,#29556,#29557,#29558,#29559,
#29560,#29561),.UNSPECIFIED.,.F.,.F.,(4,3,4),(76.7073031473017,76.9357377747032,
77.4320973732496),.UNSPECIFIED.);
#654=B_SPLINE_CURVE_WITH_KNOTS('',3,(#29564,#29565,#29566,#29567,#29568,
#29569,#29570,#29571,#29572,#29573,#29574,#29575,#29576,#29577,#29578,#29579),
 .UNSPECIFIED.,.F.,.F.,(4,3,3,3,3,4),(-75.398223686155,-74.9502993805173,
-74.4539397819708,-73.9575801834243,-73.4612205848779,-72.9814252585133),
 .UNSPECIFIED.);
#655=B_SPLINE_CURVE_WITH_KNOTS('',3,(#29585,#29586,#29587,#29588,#29589,
#29590,#29591,#29592,#29593,#29594,#29595,#29596),.UNSPECIFIED.,.F.,.F.,
(4,1,1,1,1,1,1,1,1,4),(84.8230016469244,85.302796973289,85.7991565718355,
86.295516170382,86.7918757689284,87.2882353674749,87.7845949660214,88.2809545645678,
88.7773141631143,89.2736737616608),.UNSPECIFIED.);
#656=B_SPLINE_CURVE_WITH_KNOTS('',3,(#29599,#29600,#29601,#29602,#29603,
#29604,#29605,#29606,#29607,#29608,#29609,#29610,#29611,#29612),
 .UNSPECIFIED.,.F.,.F.,(4,1,1,1,1,1,1,1,1,1,1,4),(84.8230016469244,84.8819468004013,
85.3783063989478,85.8746659974943,86.3710255960407,86.8673851945872,87.3637447931337,
87.8601043916802,88.3564639902266,88.8528235887731,89.3491831873196,89.7971074929573),
 .UNSPECIFIED.);
#657=B_SPLINE_CURVE_WITH_KNOTS('',3,(#29617,#29618,#29619,#29620,#29621,
#29622,#29623,#29624,#29625,#29626,#29627,#29628,#29629,#29630,#29631,#29632,
#29633),.UNSPECIFIED.,.F.,.F.,(4,1,1,1,1,1,1,1,1,1,1,1,1,1,4),(78.5398163397448,
78.8501221921849,79.3464817907313,79.8428413892778,80.3392009878243,80.8355605863708,
81.3319201849172,81.8282797834637,82.3246393820102,82.8209989805567,83.3173585791031,
83.8137181776496,84.3100777761961,84.8064373747425,84.8230016469244),
 .UNSPECIFIED.);
#658=B_SPLINE_CURVE_WITH_KNOTS('',3,(#29634,#29635,#29636,#29637,#29638,
#29639,#29640,#29641,#29642,#29643,#29644,#29645,#29646,#29647,#29648,#29649),
 .UNSPECIFIED.,.F.,.F.,(4,1,1,1,1,1,1,1,1,1,1,1,1,4),(78.5398163397448,
78.9256316178437,79.4219912163901,79.9183508149366,80.4147104134831,80.9110700120296,
81.407429610576,81.9037892091225,82.400148807669,82.8965084062154,83.3928680047619,
83.8892276033084,84.3855872018549,84.8230016469244),.UNSPECIFIED.);
#659=B_SPLINE_CURVE_WITH_KNOTS('',3,(#29654,#29655,#29656,#29657,#29658,
#29659,#29660,#29661,#29662,#29663,#29664,#29665,#29666,#29667,#29668,#29669,
#29670),.UNSPECIFIED.,.F.,.F.,(4,1,1,1,1,1,1,1,1,1,1,1,1,1,4),(72.2566310325652,
72.3974474110807,72.8938070096272,73.3901666081737,73.8865262067201,74.3828858052666,
74.8792454038131,75.3756050023596,75.871964600906,76.3683241994525,76.864683797999,
77.3610433965455,77.8574029950919,78.3537625936384,78.5398163397448),
 .UNSPECIFIED.);
#660=B_SPLINE_CURVE_WITH_KNOTS('',3,(#29671,#29672,#29673,#29674,#29675,
#29676,#29677,#29678,#29679,#29680,#29681,#29682,#29683,#29684,#29685,#29686,
#29687),.UNSPECIFIED.,.F.,.F.,(4,1,1,1,1,1,1,1,1,1,1,1,1,1,4),(72.2566310325652,
72.4729568367395,72.969316435286,73.4656760338325,73.9620356323789,74.4583952309254,
74.9547548294719,75.4511144280183,75.9474740265648,76.4438336251113,76.9401932236578,
77.4365528222042,77.9329124207507,78.4292720192972,78.5398163397448),
 .UNSPECIFIED.);
#661=B_SPLINE_CURVE_WITH_KNOTS('',3,(#29692,#29693,#29694,#29695,#29696,
#29697,#29698,#29699,#29700,#29701,#29702,#29703,#29704,#29705,#29706,#29707),
 .UNSPECIFIED.,.F.,.F.,(4,1,1,1,1,1,1,1,1,1,1,1,1,4),(65.9734457253856,
66.4411322285231,66.9374918270696,67.433851425616,67.9302110241625,68.426570622709,
68.9229302212554,69.4192898198019,69.9156494183484,70.4120090168948,70.9083686154413,
71.4047282139878,71.9010878125343,72.2566310325652),.UNSPECIFIED.);
#662=B_SPLINE_CURVE_WITH_KNOTS('',3,(#29708,#29709,#29710,#29711,#29712,
#29713,#29714,#29715,#29716,#29717,#29718,#29719,#29720,#29721,#29722,#29723,
#29724),.UNSPECIFIED.,.F.,.F.,(4,1,1,1,1,1,1,1,1,1,1,1,1,1,4),(65.9734457253856,
66.0202820556354,66.5166416541819,67.0130012527283,67.5093608512748,68.0057204498213,
68.5020800483677,68.9984396469142,69.4947992454607,69.9911588440072,70.4875184425536,
70.9838780411001,71.4802376396466,71.9765972381931,72.2566310325652),
 .UNSPECIFIED.);
#663=B_SPLINE_CURVE_WITH_KNOTS('',3,(#29729,#29730,#29731,#29732,#29733,
#29734,#29735,#29736,#29737,#29738,#29739,#29740,#29741,#29742,#29743,#29744,
#29745),.UNSPECIFIED.,.F.,.F.,(4,1,1,1,1,1,1,1,1,1,1,1,1,1,4),(59.690260418206,
59.9884574474189,60.4848170459654,60.9811766445119,61.4775362430584,61.9738958416048,
62.4702554401513,62.9666150386978,63.4629746372442,63.9593342357907,64.4556938343372,
64.9520534328837,65.4484130314301,65.9447726299766,65.9734457253856),
 .UNSPECIFIED.);
#664=B_SPLINE_CURVE_WITH_KNOTS('',3,(#29746,#29747,#29748,#29749,#29750,
#29751,#29752,#29753,#29754,#29755,#29756,#29757,#29758,#29759,#29760,#29761),
 .UNSPECIFIED.,.F.,.F.,(4,1,1,1,1,1,1,1,1,1,1,1,1,4),(59.690260418206,60.0639668730777,
60.5603264716242,61.0566860701707,61.5530456687171,62.0494052672636,62.5457648658101,
63.0421244643565,63.538484062903,64.0348436614495,64.531203259996,65.0275628585424,
65.5239224570889,65.9734457253856),.UNSPECIFIED.);
#665=B_SPLINE_CURVE_WITH_KNOTS('',3,(#29766,#29767,#29768,#29769,#29770,
#29771,#29772,#29773,#29774,#29775,#29776,#29777,#29778,#29779,#29780,#29781,
#29782),.UNSPECIFIED.,.F.,.F.,(4,1,1,1,1,1,1,1,1,1,1,1,1,1,4),(53.4070751110265,
53.5357826663148,54.0321422648613,54.5285018634077,55.0248614619542,55.5212210605007,
56.0175806590472,56.5139402575936,57.0102998561401,57.5066594546866,58.003019053233,
58.4993786517795,58.995738250326,59.4920978488725,59.690260418206),
 .UNSPECIFIED.);
#666=B_SPLINE_CURVE_WITH_KNOTS('',3,(#29783,#29784,#29785,#29786,#29787,
#29788,#29789,#29790,#29791,#29792,#29793,#29794,#29795,#29796,#29797,#29798,
#29799),.UNSPECIFIED.,.F.,.F.,(4,1,1,1,1,1,1,1,1,1,1,1,1,1,4),(53.4070751110264,
53.6112920919736,54.1076516905201,54.6040112890665,55.100370887613,55.5967304861595,
56.0930900847059,56.5894496832524,57.0858092817989,57.5821688803454,58.0785284788918,
58.5748880774383,59.0712476759848,59.5676072745312,59.690260418206),
 .UNSPECIFIED.);
#667=B_SPLINE_CURVE_WITH_KNOTS('',3,(#29804,#29805,#29806,#29807,#29808,
#29809,#29810,#29811,#29812,#29813,#29814,#29815,#29816,#29817,#29818,#29819),
 .UNSPECIFIED.,.F.,.F.,(4,1,1,1,1,1,1,1,1,1,1,1,1,4),(47.1238898038468,
47.5794674837571,48.0758270823036,48.5721866808501,49.0685462793965,49.564905877943,
50.0612654764895,50.557625075036,51.0539846735824,51.5503442721289,52.0467038706754,
52.5430634692219,53.0394230677683,53.4070751110265),.UNSPECIFIED.);
#668=B_SPLINE_CURVE_WITH_KNOTS('',3,(#29820,#29821,#29822,#29823,#29824,
#29825,#29826,#29827,#29828,#29829,#29830,#29831,#29832,#29833,#29834,#29835,
#29836),.UNSPECIFIED.,.F.,.F.,(4,1,1,1,1,1,1,1,1,1,1,1,1,1,4),(47.1238898038469,
47.1586173108694,47.6549769094159,48.1513365079624,48.6476961065089,49.1440557050553,
49.6404153036018,50.1367749021483,50.6331345006947,51.1294940992412,51.6258536977877,
52.1222132963342,52.6185728948806,53.1149324934271,53.4070751110264),
 .UNSPECIFIED.);
#669=B_SPLINE_CURVE_WITH_KNOTS('',3,(#29841,#29842,#29843,#29844,#29845,
#29846,#29847,#29848,#29849,#29850,#29851,#29852,#29853,#29854,#29855,#29856,
#29857),.UNSPECIFIED.,.F.,.F.,(4,1,1,1,1,1,1,1,1,1,1,1,1,1,4),(40.8407044966672,
41.126792702653,41.6231523011995,42.1195118997459,42.6158714982924,43.1122310968389,
43.6085906953854,44.1049502939318,44.6013098924783,45.0976694910248,45.5940290895712,
46.0903886881177,46.5867482866642,47.0831078852107,47.1238898038468),
 .UNSPECIFIED.);
#670=B_SPLINE_CURVE_WITH_KNOTS('',3,(#29858,#29859,#29860,#29861,#29862,
#29863,#29864,#29865,#29866,#29867,#29868,#29869,#29870,#29871,#29872,#29873),
 .UNSPECIFIED.,.F.,.F.,(4,1,1,1,1,1,1,1,1,1,1,1,1,4),(40.8407044966673,
41.2023021283118,41.6986617268582,42.1950213254047,42.6913809239512,43.1877405224977,
43.6841001210441,44.1804597195906,44.6768193181371,45.1731789166836,45.66953851523,
46.1658981137765,46.662257712323,47.1238898038469),.UNSPECIFIED.);
#671=B_SPLINE_CURVE_WITH_KNOTS('',3,(#29878,#29879,#29880,#29881,#29882,
#29883,#29884,#29885,#29886,#29887,#29888,#29889,#29890,#29891,#29892,#29893,
#29894),.UNSPECIFIED.,.F.,.F.,(4,1,1,1,1,1,1,1,1,1,1,1,1,1,4),(34.5575191894877,
34.6741179215489,35.1704775200953,35.6668371186418,36.1631967171883,36.6595563157347,
37.1559159142812,37.6522755128277,38.1486351113742,38.6449947099206,39.1413543084671,
39.6377139070136,40.1340735055601,40.6304331041065,40.8407044966672),
 .UNSPECIFIED.);
#672=B_SPLINE_CURVE_WITH_KNOTS('',3,(#29895,#29896,#29897,#29898,#29899,
#29900,#29901,#29902,#29903,#29904,#29905,#29906,#29907,#29908,#29909,#29910,
#29911),.UNSPECIFIED.,.F.,.F.,(4,1,1,1,1,1,1,1,1,1,1,1,1,1,4),(34.5575191894877,
34.7496273472076,35.2459869457541,35.7423465443006,36.2387061428471,36.7350657413935,
37.23142533994,37.7277849384865,38.2241445370329,38.7205041355794,39.2168637341259,
39.7132233326724,40.2095829312188,40.7059425297653,40.8407044966673),
 .UNSPECIFIED.);
#673=B_SPLINE_CURVE_WITH_KNOTS('',3,(#29916,#29917,#29918,#29919,#29920,
#29921,#29922,#29923,#29924,#29925,#29926,#29927,#29928,#29929,#29930,#29931),
 .UNSPECIFIED.,.F.,.F.,(4,1,1,1,1,1,1,1,1,1,1,1,1,4),(28.2743338823081,
28.7178027389912,29.2141623375377,29.7105219360841,30.2068815346306,30.7032411331771,
31.1996007317236,31.69596033027,32.1923199288165,32.688679527363,33.1850391259094,
33.6813987244559,34.1777583230024,34.5575191894877),.UNSPECIFIED.);
#674=B_SPLINE_CURVE_WITH_KNOTS('',3,(#29932,#29933,#29934,#29935,#29936,
#29937,#29938,#29939,#29940,#29941,#29942,#29943,#29944,#29945,#29946,#29947,
#29948),.UNSPECIFIED.,.F.,.F.,(4,1,1,1,1,1,1,1,1,1,1,1,1,1,4),(28.2743338823081,
28.2969525661035,28.79331216465,29.2896717631964,29.7860313617429,30.2823909602894,
30.7787505588359,31.2751101573823,31.7714697559288,32.2678293544753,32.7641889530218,
33.2605485515682,33.7569081501147,34.2532677486612,34.5575191894877),
 .UNSPECIFIED.);
#675=B_SPLINE_CURVE_WITH_KNOTS('',3,(#29953,#29954,#29955,#29956,#29957,
#29958,#29959,#29960,#29961,#29962,#29963,#29964,#29965,#29966,#29967,#29968,
#29969),.UNSPECIFIED.,.F.,.F.,(4,1,1,1,1,1,1,1,1,1,1,1,1,1,4),(21.9911485751285,
22.2651279578871,22.7614875564335,23.25784715498,23.7542067535265,24.2505663520729,
24.7469259506194,25.2432855491659,25.7396451477124,26.2360047462588,26.7323643448053,
27.2287239433518,27.7250835418983,28.2214431404447,28.2743338823081),
 .UNSPECIFIED.);
#676=B_SPLINE_CURVE_WITH_KNOTS('',3,(#29970,#29971,#29972,#29973,#29974,
#29975,#29976,#29977,#29978,#29979,#29980,#29981,#29982,#29983,#29984,#29985),
 .UNSPECIFIED.,.F.,.F.,(4,1,1,1,1,1,1,1,1,1,1,1,1,4),(21.9911485751285,
22.3406373835458,22.8369969820923,23.3333565806388,23.8297161791853,24.3260757777317,
24.8224353762782,25.3187949748247,25.8151545733711,26.3115141719176,26.8078737704641,
27.3042333690106,27.800592967557,28.2743338823081),.UNSPECIFIED.);
#677=B_SPLINE_CURVE_WITH_KNOTS('',3,(#29991,#29992,#29993,#29994,#29995,
#29996),.UNSPECIFIED.,.F.,.F.,(4,1,1,4),(14.3988838068023,14.8952434053488,
15.3916030038952,15.7079632679489),.UNSPECIFIED.);
#678=B_SPLINE_CURVE_WITH_KNOTS('',3,(#29999,#30000,#30001,#30002,#30003,
#30004,#30005),.UNSPECIFIED.,.F.,.F.,(4,1,1,1,4),(13.8754500755058,14.3233743811435,
14.81973397969,15.3160935782364,15.7079632679489),.UNSPECIFIED.);
#679=B_SPLINE_CURVE_WITH_KNOTS('',3,(#30007,#30008,#30009,#30010,#30011,
#30012,#30013,#30014,#30015,#30016,#30017,#30018,#30019,#30020,#30021,#30022,
#30023),.UNSPECIFIED.,.F.,.F.,(4,1,1,1,1,1,1,1,1,1,1,1,1,1,4),(15.7079632679489,
15.8124531767829,16.3088127753294,16.8051723738759,17.3015319724223,17.7978915709688,
18.2942511695153,18.7906107680618,19.2869703666082,19.7833299651547,20.2796895637012,
20.7760491622476,21.2724087607941,21.7687683593406,21.9911485751285),
 .UNSPECIFIED.);
#680=B_SPLINE_CURVE_WITH_KNOTS('',3,(#30024,#30025,#30026,#30027,#30028,
#30029,#30030,#30031,#30032,#30033,#30034,#30035,#30036,#30037,#30038,#30039,
#30040),.UNSPECIFIED.,.F.,.F.,(4,1,1,1,1,1,1,1,1,1,1,1,1,1,4),(15.7079632679489,
15.8879626024417,16.3843222009882,16.8806817995346,17.3770413980811,17.8734009966276,
18.3697605951741,18.8661201937205,19.362479792267,19.8588393908135,20.3551989893599,
20.8515585879064,21.3479181864529,21.8442777849994,21.9911485751285),
 .UNSPECIFIED.);
#681=B_SPLINE_CURVE_WITH_KNOTS('',3,(#30677,#30678,#30679,#30680,#30681,
#30682,#30683,#30684,#30685,#30686,#30687,#30688,#30689,#30690,#30691,#30692,
#30693,#30694,#30695,#30696,#30697,#30698,#30699,#30700,#30701,#30702,#30703,
#30704,#30705,#30706,#30707,#30708,#30709,#30710,#30711,#30712,#30713,#30714,
#30715,#30716,#30717,#30718,#30719,#30720,#30721,#30722,#30723,#30724,#30725,
#30726,#30727,#30728,#30729,#30730,#30731,#30732,#30733,#30734,#30735,#30736,
#30737,#30738,#30739,#30740,#30741,#30742,#30743,#30744,#30745,#30746,#30747,
#30748,#30749,#30750,#30751,#30752,#30753,#30754,#30755,#30756,#30757,#30758,
#30759,#30760,#30761,#30762,#30763,#30764,#30765,#30766,#30767,#30768,#30769,
#30770,#30771,#30772,#30773,#30774,#30775,#30776,#30777,#30778,#30779,#30780,
#30781,#30782,#30783,#30784,#30785,#30786,#30787,#30788,#30789,#30790,#30791,
#30792,#30793,#30794),.UNSPECIFIED.,.F.,.F.,(4,3,3,3,3,3,3,3,3,3,3,3,3,
3,3,3,3,3,3,3,3,3,3,3,3,3,3,3,3,3,3,3,3,3,3,3,3,3,3,4),(0.,0.0741055703209817,
0.149042386837593,0.22431310048934,0.299024282623367,0.348898308601355,
0.386899824489537,0.397140150473765,0.471842661155879,0.498520386535318,
0.573008003563107,0.64782102937255,0.722388891944134,0.756126730638512,
0.773706375489234,0.785503175786165,0.859722753314182,0.93387483248313,
0.992291601499154,1.0666323863286,1.11842843879762,1.14419898358481,1.16194416695704,
1.17045593848397,1.24384647704758,1.31776148692053,1.39143934948928,1.46416752858594,
1.48100080608073,1.54133664964938,1.55357748542717,1.62672847250257,1.70016992001151,
1.76604932866612,1.77729599120305,1.78733100079922,1.86043957741219,1.93296531556185,
1.96368755462996,2.01048691722679),.UNSPECIFIED.);
#682=B_SPLINE_CURVE_WITH_KNOTS('',3,(#30795,#30796,#30797,#30798,#30799,
#30800,#30801,#30802,#30803,#30804,#30805,#30806,#30807,#30808,#30809,#30810,
#30811,#30812,#30813,#30814,#30815,#30816,#30817,#30818,#30819,#30820,#30821,
#30822,#30823,#30824,#30825,#30826,#30827,#30828,#30829,#30830,#30831,#30832,
#30833,#30834,#30835,#30836,#30837,#30838,#30839,#30840,#30841,#30842,#30843,
#30844,#30845,#30846,#30847,#30848,#30849,#30850,#30851,#30852,#30853,#30854,
#30855,#30856,#30857,#30858,#30859,#30860,#30861,#30862,#30863,#30864,#30865,
#30866,#30867,#30868,#30869,#30870,#30871,#30872,#30873,#30874,#30875,#30876,
#30877,#30878,#30879,#30880,#30881,#30882,#30883,#30884,#30885,#30886,#30887,
#30888,#30889,#30890,#30891,#30892,#30893,#30894,#30895,#30896,#30897,#30898,
#30899,#30900,#30901,#30902,#30903,#30904,#30905,#30906,#30907,#30908,#30909,
#30910,#30911,#30912,#30913,#30914,#30915),.UNSPECIFIED.,.F.,.F.,(4,3,3,
3,3,3,3,3,3,3,3,3,3,3,3,3,3,3,3,3,3,3,3,3,3,3,3,3,3,3,3,3,3,3,3,3,3,3,3,
3,4),(0.,0.0717333891578521,0.144434524784762,0.217681915638706,0.290732086867526,
0.338695801228598,0.3585952673969,0.371352699087487,0.37922575171661,0.452863071133944,
0.482586944311812,0.555696925706304,0.629354906824166,0.703026073008598,
0.736450321070254,0.753797084226665,0.764865100699128,0.838737800631782,
0.912894416882333,0.970420057501849,1.04449202061033,1.09683033801563,1.12306068482966,
1.14298639667138,1.15119020265998,1.22496157430685,1.29957989448712,1.37416452133182,
1.44802364319018,1.46319855985276,1.52529555501938,1.53710295111153,1.61136302920978,
1.68616208034702,1.7546151905567,1.76661170976244,1.77674419461876,1.85186181207957,
1.92670088998344,1.95997452118572,2.00868916811693),.UNSPECIFIED.);
#683=B_SPLINE_CURVE_WITH_KNOTS('',3,(#30916,#30917,#30918,#30919,#30920,
#30921,#30922,#30923,#30924,#30925,#30926,#30927,#30928,#30929,#30930,#30931,
#30932,#30933,#30934,#30935,#30936,#30937,#30938,#30939,#30940,#30941,#30942,
#30943,#30944,#30945,#30946,#30947,#30948,#30949,#30950,#30951,#30952,#30953,
#30954,#30955,#30956,#30957,#30958),.UNSPECIFIED.,.F.,.F.,(4,3,3,3,3,3,
3,3,3,3,3,3,3,3,4),(-72.9814252585133,-72.9648609863314,-72.4685013877849,
-71.9721417892385,-71.475782190692,-70.9794225921455,-70.483062993599,-69.9867033950526,
-69.4903437965061,-68.9939841979596,-68.4976245994131,-68.0012650008667,
-67.5049054023202,-67.0085458037737,-66.6982399513337),.UNSPECIFIED.);
#684=B_SPLINE_CURVE_WITH_KNOTS('',3,(#31595,#31596,#31597,#31598,#31599,
#31600,#31601,#31602,#31603,#31604,#31605,#31606,#31607,#31608,#31609,#31610,
#31611,#31612,#31613,#31614,#31615,#31616,#31617,#31618,#31619,#31620,#31621,
#31622,#31623,#31624,#31625,#31626,#31627,#31628,#31629,#31630,#31631,#31632,
#31633,#31634,#31635,#31636,#31637,#31638,#31639,#31640,#31641,#31642,#31643,
#31644,#31645,#31646,#31647,#31648,#31649,#31650,#31651,#31652,#31653,#31654,
#31655,#31656,#31657,#31658,#31659,#31660,#31661,#31662,#31663,#31664,#31665,
#31666,#31667,#31668,#31669,#31670,#31671,#31672,#31673,#31674,#31675,#31676,
#31677,#31678,#31679,#31680,#31681,#31682,#31683,#31684,#31685,#31686,#31687,
#31688,#31689,#31690,#31691,#31692,#31693,#31694,#31695,#31696,#31697,#31698,
#31699,#31700,#31701,#31702,#31703,#31704,#31705,#31706,#31707,#31708,#31709,
#31710,#31711,#31712,#31713,#31714,#31715),.UNSPECIFIED.,.F.,.F.,(4,3,3,
3,3,3,3,3,3,3,3,3,3,3,3,3,3,3,3,3,3,3,3,3,3,3,3,3,3,3,3,3,3,3,3,3,3,3,3,
3,4),(0.,0.0717334165710816,0.14443457078409,0.217681968816114,0.290732129582985,
0.338695833265186,0.358595323769131,0.371352811334654,0.379225821480966,
0.452863145034527,0.482586944311789,0.555696909117683,0.629354883241453,
0.703026051028594,0.736450301837749,0.75379706834374,0.764865101436399,
0.838737791296975,0.91289440941722,0.970420057501839,1.044492023981,1.09683034096497,
1.1230606915887,1.14298630277634,1.15119019060978,1.2249615711206,1.29957989345465,
1.37416452034083,1.44802364240076,1.46319855985276,1.52529555501938,1.53710295132795,
1.61136302929257,1.68616208097367,1.75461519102668,1.7666117106576,1.77674419560174,
1.85186181352304,1.9267008900023,1.95997452118571,2.00868916811694),
 .UNSPECIFIED.);
#685=B_SPLINE_CURVE_WITH_KNOTS('',3,(#31716,#31717,#31718,#31719,#31720,
#31721,#31722,#31723,#31724,#31725,#31726,#31727,#31728,#31729,#31730,#31731,
#31732,#31733,#31734,#31735,#31736,#31737,#31738,#31739,#31740,#31741,#31742,
#31743,#31744,#31745,#31746,#31747,#31748,#31749,#31750,#31751,#31752,#31753,
#31754,#31755,#31756,#31757,#31758),.UNSPECIFIED.,.F.,.F.,(4,3,3,3,3,3,
3,3,3,3,3,3,3,3,4),(70.4241178401221,70.483062993599,70.9794225921455,71.475782190692,
71.9721417892384,72.4685013877849,72.9648609863314,73.4612205848779,73.9575801834243,
74.4539397819708,74.9502993805173,75.4466589790638,75.9430185776102,76.4393781761567,
76.7073031473017),.UNSPECIFIED.);
#686=B_SPLINE_CURVE_WITH_KNOTS('',3,(#31759,#31760,#31761,#31762,#31763,
#31764,#31765,#31766,#31767,#31768,#31769,#31770,#31771,#31772,#31773,#31774,
#31775,#31776,#31777,#31778,#31779,#31780,#31781,#31782,#31783,#31784,#31785,
#31786,#31787,#31788,#31789,#31790,#31791,#31792,#31793,#31794,#31795,#31796,
#31797,#31798,#31799,#31800,#31801,#31802,#31803,#31804,#31805,#31806,#31807,
#31808,#31809,#31810,#31811,#31812,#31813,#31814,#31815,#31816,#31817,#31818,
#31819,#31820,#31821,#31822,#31823,#31824,#31825,#31826,#31827,#31828,#31829,
#31830,#31831,#31832,#31833,#31834,#31835,#31836,#31837,#31838,#31839,#31840,
#31841,#31842,#31843,#31844,#31845,#31846,#31847,#31848,#31849,#31850,#31851,
#31852,#31853,#31854,#31855,#31856,#31857,#31858,#31859,#31860,#31861,#31862,
#31863,#31864,#31865,#31866,#31867,#31868,#31869,#31870,#31871,#31872,#31873,
#31874,#31875,#31876),.UNSPECIFIED.,.F.,.F.,(4,3,3,3,3,3,3,3,3,3,3,3,3,
3,3,3,3,3,3,3,3,3,3,3,3,3,3,3,3,3,3,3,3,3,3,3,3,3,3,4),(0.,0.0741055943583196,
0.149042424272304,0.224313139225513,0.299024306861181,0.348898326779717,
0.3868998616391,0.397140157099964,0.471842665351292,0.498520386535326,0.573007992260638,
0.647821015783437,0.722388882730898,0.756126722576926,0.773706368904776,
0.78550317616495,0.859722748844764,0.93387483251693,0.992291601499126,1.06663238757372,
1.1184284398871,1.1441989874156,1.16194405544069,1.17045593148218,1.24384647547351,
1.31776148594777,1.39143934859838,1.46416752984131,1.48100080608075,1.5413366496494,
1.55357748570526,1.62672847367446,1.70016992167766,1.76604932991573,1.77729599482936,
1.78733100568737,1.86043958226664,1.93296531739482,1.96368755462995,2.01048691722678),
 .UNSPECIFIED.);
#1028=CONICAL_SURFACE('',#18638,13.3,0.785398163397449);
#1462=FACE_BOUND('',#4028,.T.);
#1463=FACE_BOUND('',#4032,.T.);
#1464=FACE_BOUND('',#4036,.T.);
#2141=CIRCLE('',#18601,9.64155);
#2142=CIRCLE('',#18613,9.64155);
#2143=CIRCLE('',#18615,10.06205);
#2144=CIRCLE('',#18627,10.06205);
#2145=CIRCLE('',#18630,12.5);
#2146=CIRCLE('',#18633,12.5);
#2147=CIRCLE('',#18635,13.5);
#2148=CIRCLE('',#18637,13.5);
#2149=CIRCLE('',#18639,13.1);
#2987=FACE_OUTER_BOUND('',#4000,.T.);
#2988=FACE_OUTER_BOUND('',#4001,.T.);
#2989=FACE_OUTER_BOUND('',#4002,.T.);
#2990=FACE_OUTER_BOUND('',#4003,.T.);
#2991=FACE_OUTER_BOUND('',#4004,.T.);
#2992=FACE_OUTER_BOUND('',#4005,.T.);
#2993=FACE_OUTER_BOUND('',#4006,.T.);
#2994=FACE_OUTER_BOUND('',#4007,.T.);
#2995=FACE_OUTER_BOUND('',#4008,.T.);
#2996=FACE_OUTER_BOUND('',#4009,.T.);
#2997=FACE_OUTER_BOUND('',#4010,.T.);
#2998=FACE_OUTER_BOUND('',#4011,.T.);
#2999=FACE_OUTER_BOUND('',#4012,.T.);
#3000=FACE_OUTER_BOUND('',#4013,.T.);
#3001=FACE_OUTER_BOUND('',#4014,.T.);
#3002=FACE_OUTER_BOUND('',#4015,.T.);
#3003=FACE_OUTER_BOUND('',#4016,.T.);
#3004=FACE_OUTER_BOUND('',#4017,.T.);
#3005=FACE_OUTER_BOUND('',#4018,.T.);
#3006=FACE_OUTER_BOUND('',#4019,.T.);
#3007=FACE_OUTER_BOUND('',#4020,.T.);
#3008=FACE_OUTER_BOUND('',#4021,.T.);
#3009=FACE_OUTER_BOUND('',#4022,.T.);
#3010=FACE_OUTER_BOUND('',#4023,.T.);
#3011=FACE_OUTER_BOUND('',#4024,.T.);
#3012=FACE_OUTER_BOUND('',#4025,.T.);
#3013=FACE_OUTER_BOUND('',#4026,.T.);
#3014=FACE_OUTER_BOUND('',#4027,.T.);
#3015=FACE_OUTER_BOUND('',#4029,.T.);
#3016=FACE_OUTER_BOUND('',#4030,.T.);
#3017=FACE_OUTER_BOUND('',#4031,.T.);
#3018=FACE_OUTER_BOUND('',#4033,.T.);
#3019=FACE_OUTER_BOUND('',#4034,.T.);
#3020=FACE_OUTER_BOUND('',#4035,.T.);
#4000=EDGE_LOOP('',(#14181,#14182,#14183,#14184));
#4001=EDGE_LOOP('',(#14185,#14186,#14187,#14188));
#4002=EDGE_LOOP('',(#14189,#14190,#14191,#14192));
#4003=EDGE_LOOP('',(#14193,#14194,#14195,#14196));
#4004=EDGE_LOOP('',(#14197,#14198,#14199,#14200));
#4005=EDGE_LOOP('',(#14201,#14202,#14203,#14204));
#4006=EDGE_LOOP('',(#14205,#14206,#14207,#14208));
#4007=EDGE_LOOP('',(#14209,#14210,#14211,#14212));
#4008=EDGE_LOOP('',(#14213,#14214,#14215,#14216));
#4009=EDGE_LOOP('',(#14217,#14218,#14219,#14220));
#4010=EDGE_LOOP('',(#14221,#14222,#14223,#14224));
#4011=EDGE_LOOP('',(#14225,#14226,#14227,#14228));
#4012=EDGE_LOOP('',(#14229,#14230,#14231,#14232));
#4013=EDGE_LOOP('',(#14233,#14234,#14235,#14236));
#4014=EDGE_LOOP('',(#14237,#14238,#14239,#14240));
#4015=EDGE_LOOP('',(#14241,#14242,#14243,#14244));
#4016=EDGE_LOOP('',(#14245,#14246,#14247,#14248));
#4017=EDGE_LOOP('',(#14249,#14250,#14251,#14252));
#4018=EDGE_LOOP('',(#14253,#14254,#14255,#14256));
#4019=EDGE_LOOP('',(#14257,#14258,#14259,#14260));
#4020=EDGE_LOOP('',(#14261,#14262,#14263,#14264));
#4021=EDGE_LOOP('',(#14265,#14266,#14267,#14268));
#4022=EDGE_LOOP('',(#14269,#14270,#14271,#14272));
#4023=EDGE_LOOP('',(#14273,#14274,#14275,#14276));
#4024=EDGE_LOOP('',(#14277,#14278,#14279,#14280));
#4025=EDGE_LOOP('',(#14281,#14282,#14283,#14284,#14285,#14286,#14287,#14288,
#14289,#14290,#14291,#14292,#14293,#14294,#14295,#14296,#14297,#14298,#14299,
#14300,#14301,#14302,#14303,#14304,#14305,#14306,#14307,#14308));
#4026=EDGE_LOOP('',(#14309,#14310,#14311,#14312,#14313,#14314,#14315,#14316,
#14317,#14318,#14319,#14320,#14321,#14322,#14323,#14324,#14325,#14326,#14327,
#14328,#14329,#14330,#14331,#14332,#14333,#14334,#14335,#14336));
#4027=EDGE_LOOP('',(#14337));
#4028=EDGE_LOOP('',(#14338,#14339,#14340,#14341));
#4029=EDGE_LOOP('',(#14342,#14343,#14344,#14345));
#4030=EDGE_LOOP('',(#14346,#14347,#14348,#14349));
#4031=EDGE_LOOP('',(#14350));
#4032=EDGE_LOOP('',(#14351));
#4033=EDGE_LOOP('',(#14352,#14353,#14354,#14355));
#4034=EDGE_LOOP('',(#14356,#14357,#14358,#14359));
#4035=EDGE_LOOP('',(#14360));
#4036=EDGE_LOOP('',(#14361,#14362,#14363,#14364));
#4977=LINE('',#28605,#5952);
#4978=LINE('',#28674,#5953);
#4979=LINE('',#28761,#5954);
#4980=LINE('',#28851,#5955);
#4981=LINE('',#28938,#5956);
#4982=LINE('',#29025,#5957);
#4983=LINE('',#29115,#5958);
#4984=LINE('',#29202,#5959);
#4985=LINE('',#29289,#5960);
#4986=LINE('',#29379,#5961);
#4987=LINE('',#29466,#5962);
#4988=LINE('',#29553,#5963);
#4989=LINE('',#29583,#5964);
#4990=LINE('',#29616,#5965);
#4991=LINE('',#29653,#5966);
#4992=LINE('',#29691,#5967);
#4993=LINE('',#29728,#5968);
#4994=LINE('',#29765,#5969);
#4995=LINE('',#29803,#5970);
#4996=LINE('',#29840,#5971);
#4997=LINE('',#29877,#5972);
#4998=LINE('',#29915,#5973);
#4999=LINE('',#29952,#5974);
#5000=LINE('',#29989,#5975);
#5001=LINE('',#31884,#5976);
#5002=LINE('',#31891,#5977);
#5003=LINE('',#31895,#5978);
#5952=VECTOR('',#22479,9.6);
#5953=VECTOR('',#22484,9.6);
#5954=VECTOR('',#22487,9.6);
#5955=VECTOR('',#22490,9.6);
#5956=VECTOR('',#22493,9.6);
#5957=VECTOR('',#22496,9.6);
#5958=VECTOR('',#22499,9.6);
#5959=VECTOR('',#22502,9.6);
#5960=VECTOR('',#22505,9.6);
#5961=VECTOR('',#22508,9.6);
#5962=VECTOR('',#22511,9.6);
#5963=VECTOR('',#22514,9.6);
#5964=VECTOR('',#22519,10.06205);
#5965=VECTOR('',#22524,10.06205);
#5966=VECTOR('',#22527,10.06205);
#5967=VECTOR('',#22530,10.06205);
#5968=VECTOR('',#22533,10.06205);
#5969=VECTOR('',#22536,10.06205);
#5970=VECTOR('',#22539,10.06205);
#5971=VECTOR('',#22542,10.06205);
#5972=VECTOR('',#22545,10.06205);
#5973=VECTOR('',#22548,10.06205);
#5974=VECTOR('',#22551,10.06205);
#5975=VECTOR('',#22554,10.06205);
#5976=VECTOR('',#22569,12.5);
#5977=VECTOR('',#22578,13.5);
#5978=VECTOR('',#22583,13.3);
#7413=VERTEX_POINT('',#28603);
#7414=VERTEX_POINT('',#28604);
#7415=VERTEX_POINT('',#28606);
#7416=VERTEX_POINT('',#28632);
#7417=VERTEX_POINT('',#28672);
#7418=VERTEX_POINT('',#28673);
#7419=VERTEX_POINT('',#28759);
#7420=VERTEX_POINT('',#28760);
#7421=VERTEX_POINT('',#28849);
#7422=VERTEX_POINT('',#28850);
#7423=VERTEX_POINT('',#28936);
#7424=VERTEX_POINT('',#28937);
#7425=VERTEX_POINT('',#29023);
#7426=VERTEX_POINT('',#29024);
#7427=VERTEX_POINT('',#29113);
#7428=VERTEX_POINT('',#29114);
#7429=VERTEX_POINT('',#29200);
#7430=VERTEX_POINT('',#29201);
#7431=VERTEX_POINT('',#29287);
#7432=VERTEX_POINT('',#29288);
#7433=VERTEX_POINT('',#29377);
#7434=VERTEX_POINT('',#29378);
#7435=VERTEX_POINT('',#29464);
#7436=VERTEX_POINT('',#29465);
#7437=VERTEX_POINT('',#29551);
#7438=VERTEX_POINT('',#29552);
#7439=VERTEX_POINT('',#29554);
#7440=VERTEX_POINT('',#29562);
#7441=VERTEX_POINT('',#29581);
#7442=VERTEX_POINT('',#29582);
#7443=VERTEX_POINT('',#29584);
#7444=VERTEX_POINT('',#29597);
#7445=VERTEX_POINT('',#29614);
#7446=VERTEX_POINT('',#29615);
#7447=VERTEX_POINT('',#29651);
#7448=VERTEX_POINT('',#29652);
#7449=VERTEX_POINT('',#29689);
#7450=VERTEX_POINT('',#29690);
#7451=VERTEX_POINT('',#29726);
#7452=VERTEX_POINT('',#29727);
#7453=VERTEX_POINT('',#29763);
#7454=VERTEX_POINT('',#29764);
#7455=VERTEX_POINT('',#29801);
#7456=VERTEX_POINT('',#29802);
#7457=VERTEX_POINT('',#29838);
#7458=VERTEX_POINT('',#29839);
#7459=VERTEX_POINT('',#29875);
#7460=VERTEX_POINT('',#29876);
#7461=VERTEX_POINT('',#29913);
#7462=VERTEX_POINT('',#29914);
#7463=VERTEX_POINT('',#29950);
#7464=VERTEX_POINT('',#29951);
#7465=VERTEX_POINT('',#29987);
#7466=VERTEX_POINT('',#29988);
#7467=VERTEX_POINT('',#29990);
#7468=VERTEX_POINT('',#29997);
#7469=VERTEX_POINT('',#31878);
#7470=VERTEX_POINT('',#31882);
#7471=VERTEX_POINT('',#31886);
#7472=VERTEX_POINT('',#31889);
#7473=VERTEX_POINT('',#31893);
#9742=EDGE_CURVE('',#7413,#7414,#4977,.T.);
#9743=EDGE_CURVE('',#7414,#7415,#631,.T.);
#9744=EDGE_CURVE('',#7416,#7415,#2141,.F.);
#9745=EDGE_CURVE('',#7416,#7413,#632,.T.);
#9746=EDGE_CURVE('',#7417,#7418,#4978,.T.);
#9747=EDGE_CURVE('',#7418,#7414,#633,.T.);
#9748=EDGE_CURVE('',#7413,#7417,#634,.T.);
#9749=EDGE_CURVE('',#7419,#7420,#4979,.T.);
#9750=EDGE_CURVE('',#7420,#7418,#635,.T.);
#9751=EDGE_CURVE('',#7417,#7419,#636,.T.);
#9752=EDGE_CURVE('',#7421,#7422,#4980,.T.);
#9753=EDGE_CURVE('',#7422,#7420,#637,.T.);
#9754=EDGE_CURVE('',#7419,#7421,#638,.T.);
#9755=EDGE_CURVE('',#7423,#7424,#4981,.T.);
#9756=EDGE_CURVE('',#7424,#7422,#639,.T.);
#9757=EDGE_CURVE('',#7421,#7423,#640,.T.);
#9758=EDGE_CURVE('',#7425,#7426,#4982,.T.);
#9759=EDGE_CURVE('',#7426,#7424,#641,.T.);
#9760=EDGE_CURVE('',#7423,#7425,#642,.T.);
#9761=EDGE_CURVE('',#7427,#7428,#4983,.T.);
#9762=EDGE_CURVE('',#7428,#7426,#643,.T.);
#9763=EDGE_CURVE('',#7425,#7427,#644,.T.);
#9764=EDGE_CURVE('',#7429,#7430,#4984,.T.);
#9765=EDGE_CURVE('',#7430,#7428,#645,.T.);
#9766=EDGE_CURVE('',#7427,#7429,#646,.T.);
#9767=EDGE_CURVE('',#7431,#7432,#4985,.T.);
#9768=EDGE_CURVE('',#7432,#7430,#647,.T.);
#9769=EDGE_CURVE('',#7429,#7431,#648,.T.);
#9770=EDGE_CURVE('',#7433,#7434,#4986,.T.);
#9771=EDGE_CURVE('',#7434,#7432,#649,.T.);
#9772=EDGE_CURVE('',#7431,#7433,#650,.T.);
#9773=EDGE_CURVE('',#7435,#7436,#4987,.T.);
#9774=EDGE_CURVE('',#7436,#7434,#651,.T.);
#9775=EDGE_CURVE('',#7433,#7435,#652,.T.);
#9776=EDGE_CURVE('',#7437,#7438,#4988,.T.);
#9777=EDGE_CURVE('',#7437,#7439,#653,.T.);
#9778=EDGE_CURVE('',#7439,#7440,#2142,.T.);
#9779=EDGE_CURVE('',#7440,#7438,#654,.T.);
#9780=EDGE_CURVE('',#7441,#7442,#4989,.T.);
#9781=EDGE_CURVE('',#7442,#7443,#655,.T.);
#9782=EDGE_CURVE('',#7444,#7443,#2143,.T.);
#9783=EDGE_CURVE('',#7441,#7444,#656,.T.);
#9784=EDGE_CURVE('',#7445,#7446,#4990,.T.);
#9785=EDGE_CURVE('',#7446,#7442,#657,.T.);
#9786=EDGE_CURVE('',#7445,#7441,#658,.T.);
#9787=EDGE_CURVE('',#7447,#7448,#4991,.T.);
#9788=EDGE_CURVE('',#7448,#7446,#659,.T.);
#9789=EDGE_CURVE('',#7447,#7445,#660,.T.);
#9790=EDGE_CURVE('',#7449,#7450,#4992,.T.);
#9791=EDGE_CURVE('',#7450,#7448,#661,.T.);
#9792=EDGE_CURVE('',#7449,#7447,#662,.T.);
#9793=EDGE_CURVE('',#7451,#7452,#4993,.T.);
#9794=EDGE_CURVE('',#7452,#7450,#663,.T.);
#9795=EDGE_CURVE('',#7451,#7449,#664,.T.);
#9796=EDGE_CURVE('',#7453,#7454,#4994,.T.);
#9797=EDGE_CURVE('',#7454,#7452,#665,.T.);
#9798=EDGE_CURVE('',#7453,#7451,#666,.T.);
#9799=EDGE_CURVE('',#7455,#7456,#4995,.T.);
#9800=EDGE_CURVE('',#7456,#7454,#667,.T.);
#9801=EDGE_CURVE('',#7455,#7453,#668,.T.);
#9802=EDGE_CURVE('',#7457,#7458,#4996,.T.);
#9803=EDGE_CURVE('',#7458,#7456,#669,.T.);
#9804=EDGE_CURVE('',#7457,#7455,#670,.T.);
#9805=EDGE_CURVE('',#7459,#7460,#4997,.T.);
#9806=EDGE_CURVE('',#7460,#7458,#671,.T.);
#9807=EDGE_CURVE('',#7459,#7457,#672,.T.);
#9808=EDGE_CURVE('',#7461,#7462,#4998,.T.);
#9809=EDGE_CURVE('',#7462,#7460,#673,.T.);
#9810=EDGE_CURVE('',#7461,#7459,#674,.T.);
#9811=EDGE_CURVE('',#7463,#7464,#4999,.T.);
#9812=EDGE_CURVE('',#7464,#7462,#675,.T.);
#9813=EDGE_CURVE('',#7463,#7461,#676,.T.);
#9814=EDGE_CURVE('',#7465,#7466,#5000,.T.);
#9815=EDGE_CURVE('',#7467,#7465,#677,.T.);
#9816=EDGE_CURVE('',#7468,#7467,#2144,.T.);
#9817=EDGE_CURVE('',#7468,#7466,#678,.T.);
#9818=EDGE_CURVE('',#7466,#7464,#679,.T.);
#9819=EDGE_CURVE('',#7465,#7463,#680,.T.);
#9820=EDGE_CURVE('',#7443,#7440,#681,.T.);
#9821=EDGE_CURVE('',#7415,#7468,#682,.T.);
#9822=EDGE_CURVE('',#7438,#7436,#683,.T.);
#9823=EDGE_CURVE('',#7439,#7444,#684,.T.);
#9824=EDGE_CURVE('',#7435,#7437,#685,.T.);
#9825=EDGE_CURVE('',#7467,#7416,#686,.T.);
#9826=EDGE_CURVE('',#7469,#7469,#2145,.T.);
#9827=EDGE_CURVE('',#7470,#7470,#2146,.T.);
#9828=EDGE_CURVE('',#7470,#7469,#5001,.T.);
#9829=EDGE_CURVE('',#7471,#7471,#2147,.T.);
#9830=EDGE_CURVE('',#7472,#7472,#2148,.T.);
#9831=EDGE_CURVE('',#7472,#7471,#5002,.T.);
#9832=EDGE_CURVE('',#7473,#7473,#2149,.T.);
#9833=EDGE_CURVE('',#7473,#7472,#5003,.T.);
#14181=ORIENTED_EDGE('',*,*,#9742,.T.);
#14182=ORIENTED_EDGE('',*,*,#9743,.T.);
#14183=ORIENTED_EDGE('',*,*,#9744,.F.);
#14184=ORIENTED_EDGE('',*,*,#9745,.T.);
#14185=ORIENTED_EDGE('',*,*,#9746,.T.);
#14186=ORIENTED_EDGE('',*,*,#9747,.T.);
#14187=ORIENTED_EDGE('',*,*,#9742,.F.);
#14188=ORIENTED_EDGE('',*,*,#9748,.T.);
#14189=ORIENTED_EDGE('',*,*,#9749,.T.);
#14190=ORIENTED_EDGE('',*,*,#9750,.T.);
#14191=ORIENTED_EDGE('',*,*,#9746,.F.);
#14192=ORIENTED_EDGE('',*,*,#9751,.T.);
#14193=ORIENTED_EDGE('',*,*,#9752,.T.);
#14194=ORIENTED_EDGE('',*,*,#9753,.T.);
#14195=ORIENTED_EDGE('',*,*,#9749,.F.);
#14196=ORIENTED_EDGE('',*,*,#9754,.T.);
#14197=ORIENTED_EDGE('',*,*,#9755,.T.);
#14198=ORIENTED_EDGE('',*,*,#9756,.T.);
#14199=ORIENTED_EDGE('',*,*,#9752,.F.);
#14200=ORIENTED_EDGE('',*,*,#9757,.T.);
#14201=ORIENTED_EDGE('',*,*,#9758,.T.);
#14202=ORIENTED_EDGE('',*,*,#9759,.T.);
#14203=ORIENTED_EDGE('',*,*,#9755,.F.);
#14204=ORIENTED_EDGE('',*,*,#9760,.T.);
#14205=ORIENTED_EDGE('',*,*,#9761,.T.);
#14206=ORIENTED_EDGE('',*,*,#9762,.T.);
#14207=ORIENTED_EDGE('',*,*,#9758,.F.);
#14208=ORIENTED_EDGE('',*,*,#9763,.T.);
#14209=ORIENTED_EDGE('',*,*,#9764,.T.);
#14210=ORIENTED_EDGE('',*,*,#9765,.T.);
#14211=ORIENTED_EDGE('',*,*,#9761,.F.);
#14212=ORIENTED_EDGE('',*,*,#9766,.T.);
#14213=ORIENTED_EDGE('',*,*,#9767,.T.);
#14214=ORIENTED_EDGE('',*,*,#9768,.T.);
#14215=ORIENTED_EDGE('',*,*,#9764,.F.);
#14216=ORIENTED_EDGE('',*,*,#9769,.T.);
#14217=ORIENTED_EDGE('',*,*,#9770,.T.);
#14218=ORIENTED_EDGE('',*,*,#9771,.T.);
#14219=ORIENTED_EDGE('',*,*,#9767,.F.);
#14220=ORIENTED_EDGE('',*,*,#9772,.T.);
#14221=ORIENTED_EDGE('',*,*,#9773,.T.);
#14222=ORIENTED_EDGE('',*,*,#9774,.T.);
#14223=ORIENTED_EDGE('',*,*,#9770,.F.);
#14224=ORIENTED_EDGE('',*,*,#9775,.T.);
#14225=ORIENTED_EDGE('',*,*,#9776,.F.);
#14226=ORIENTED_EDGE('',*,*,#9777,.T.);
#14227=ORIENTED_EDGE('',*,*,#9778,.T.);
#14228=ORIENTED_EDGE('',*,*,#9779,.T.);
#14229=ORIENTED_EDGE('',*,*,#9780,.T.);
#14230=ORIENTED_EDGE('',*,*,#9781,.T.);
#14231=ORIENTED_EDGE('',*,*,#9782,.F.);
#14232=ORIENTED_EDGE('',*,*,#9783,.F.);
#14233=ORIENTED_EDGE('',*,*,#9784,.T.);
#14234=ORIENTED_EDGE('',*,*,#9785,.T.);
#14235=ORIENTED_EDGE('',*,*,#9780,.F.);
#14236=ORIENTED_EDGE('',*,*,#9786,.F.);
#14237=ORIENTED_EDGE('',*,*,#9787,.T.);
#14238=ORIENTED_EDGE('',*,*,#9788,.T.);
#14239=ORIENTED_EDGE('',*,*,#9784,.F.);
#14240=ORIENTED_EDGE('',*,*,#9789,.F.);
#14241=ORIENTED_EDGE('',*,*,#9790,.T.);
#14242=ORIENTED_EDGE('',*,*,#9791,.T.);
#14243=ORIENTED_EDGE('',*,*,#9787,.F.);
#14244=ORIENTED_EDGE('',*,*,#9792,.F.);
#14245=ORIENTED_EDGE('',*,*,#9793,.T.);
#14246=ORIENTED_EDGE('',*,*,#9794,.T.);
#14247=ORIENTED_EDGE('',*,*,#9790,.F.);
#14248=ORIENTED_EDGE('',*,*,#9795,.F.);
#14249=ORIENTED_EDGE('',*,*,#9796,.T.);
#14250=ORIENTED_EDGE('',*,*,#9797,.T.);
#14251=ORIENTED_EDGE('',*,*,#9793,.F.);
#14252=ORIENTED_EDGE('',*,*,#9798,.F.);
#14253=ORIENTED_EDGE('',*,*,#9799,.T.);
#14254=ORIENTED_EDGE('',*,*,#9800,.T.);
#14255=ORIENTED_EDGE('',*,*,#9796,.F.);
#14256=ORIENTED_EDGE('',*,*,#9801,.F.);
#14257=ORIENTED_EDGE('',*,*,#9802,.T.);
#14258=ORIENTED_EDGE('',*,*,#9803,.T.);
#14259=ORIENTED_EDGE('',*,*,#9799,.F.);
#14260=ORIENTED_EDGE('',*,*,#9804,.F.);
#14261=ORIENTED_EDGE('',*,*,#9805,.T.);
#14262=ORIENTED_EDGE('',*,*,#9806,.T.);
#14263=ORIENTED_EDGE('',*,*,#9802,.F.);
#14264=ORIENTED_EDGE('',*,*,#9807,.F.);
#14265=ORIENTED_EDGE('',*,*,#9808,.T.);
#14266=ORIENTED_EDGE('',*,*,#9809,.T.);
#14267=ORIENTED_EDGE('',*,*,#9805,.F.);
#14268=ORIENTED_EDGE('',*,*,#9810,.F.);
#14269=ORIENTED_EDGE('',*,*,#9811,.T.);
#14270=ORIENTED_EDGE('',*,*,#9812,.T.);
#14271=ORIENTED_EDGE('',*,*,#9808,.F.);
#14272=ORIENTED_EDGE('',*,*,#9813,.F.);
#14273=ORIENTED_EDGE('',*,*,#9814,.F.);
#14274=ORIENTED_EDGE('',*,*,#9815,.F.);
#14275=ORIENTED_EDGE('',*,*,#9816,.F.);
#14276=ORIENTED_EDGE('',*,*,#9817,.T.);
#14277=ORIENTED_EDGE('',*,*,#9814,.T.);
#14278=ORIENTED_EDGE('',*,*,#9818,.T.);
#14279=ORIENTED_EDGE('',*,*,#9811,.F.);
#14280=ORIENTED_EDGE('',*,*,#9819,.F.);
#14281=ORIENTED_EDGE('',*,*,#9820,.F.);
#14282=ORIENTED_EDGE('',*,*,#9781,.F.);
#14283=ORIENTED_EDGE('',*,*,#9785,.F.);
#14284=ORIENTED_EDGE('',*,*,#9788,.F.);
#14285=ORIENTED_EDGE('',*,*,#9791,.F.);
#14286=ORIENTED_EDGE('',*,*,#9794,.F.);
#14287=ORIENTED_EDGE('',*,*,#9797,.F.);
#14288=ORIENTED_EDGE('',*,*,#9800,.F.);
#14289=ORIENTED_EDGE('',*,*,#9803,.F.);
#14290=ORIENTED_EDGE('',*,*,#9806,.F.);
#14291=ORIENTED_EDGE('',*,*,#9809,.F.);
#14292=ORIENTED_EDGE('',*,*,#9812,.F.);
#14293=ORIENTED_EDGE('',*,*,#9818,.F.);
#14294=ORIENTED_EDGE('',*,*,#9817,.F.);
#14295=ORIENTED_EDGE('',*,*,#9821,.F.);
#14296=ORIENTED_EDGE('',*,*,#9743,.F.);
#14297=ORIENTED_EDGE('',*,*,#9747,.F.);
#14298=ORIENTED_EDGE('',*,*,#9750,.F.);
#14299=ORIENTED_EDGE('',*,*,#9753,.F.);
#14300=ORIENTED_EDGE('',*,*,#9756,.F.);
#14301=ORIENTED_EDGE('',*,*,#9759,.F.);
#14302=ORIENTED_EDGE('',*,*,#9762,.F.);
#14303=ORIENTED_EDGE('',*,*,#9765,.F.);
#14304=ORIENTED_EDGE('',*,*,#9768,.F.);
#14305=ORIENTED_EDGE('',*,*,#9771,.F.);
#14306=ORIENTED_EDGE('',*,*,#9774,.F.);
#14307=ORIENTED_EDGE('',*,*,#9822,.F.);
#14308=ORIENTED_EDGE('',*,*,#9779,.F.);
#14309=ORIENTED_EDGE('',*,*,#9823,.F.);
#14310=ORIENTED_EDGE('',*,*,#9777,.F.);
#14311=ORIENTED_EDGE('',*,*,#9824,.F.);
#14312=ORIENTED_EDGE('',*,*,#9775,.F.);
#14313=ORIENTED_EDGE('',*,*,#9772,.F.);
#14314=ORIENTED_EDGE('',*,*,#9769,.F.);
#14315=ORIENTED_EDGE('',*,*,#9766,.F.);
#14316=ORIENTED_EDGE('',*,*,#9763,.F.);
#14317=ORIENTED_EDGE('',*,*,#9760,.F.);
#14318=ORIENTED_EDGE('',*,*,#9757,.F.);
#14319=ORIENTED_EDGE('',*,*,#9754,.F.);
#14320=ORIENTED_EDGE('',*,*,#9751,.F.);
#14321=ORIENTED_EDGE('',*,*,#9748,.F.);
#14322=ORIENTED_EDGE('',*,*,#9745,.F.);
#14323=ORIENTED_EDGE('',*,*,#9825,.F.);
#14324=ORIENTED_EDGE('',*,*,#9815,.T.);
#14325=ORIENTED_EDGE('',*,*,#9819,.T.);
#14326=ORIENTED_EDGE('',*,*,#9813,.T.);
#14327=ORIENTED_EDGE('',*,*,#9810,.T.);
#14328=ORIENTED_EDGE('',*,*,#9807,.T.);
#14329=ORIENTED_EDGE('',*,*,#9804,.T.);
#14330=ORIENTED_EDGE('',*,*,#9801,.T.);
#14331=ORIENTED_EDGE('',*,*,#9798,.T.);
#14332=ORIENTED_EDGE('',*,*,#9795,.T.);
#14333=ORIENTED_EDGE('',*,*,#9792,.T.);
#14334=ORIENTED_EDGE('',*,*,#9789,.T.);
#14335=ORIENTED_EDGE('',*,*,#9786,.T.);
#14336=ORIENTED_EDGE('',*,*,#9783,.T.);
#14337=ORIENTED_EDGE('',*,*,#9826,.F.);
#14338=ORIENTED_EDGE('',*,*,#9821,.T.);
#14339=ORIENTED_EDGE('',*,*,#9816,.T.);
#14340=ORIENTED_EDGE('',*,*,#9825,.T.);
#14341=ORIENTED_EDGE('',*,*,#9744,.T.);
#14342=ORIENTED_EDGE('',*,*,#9776,.T.);
#14343=ORIENTED_EDGE('',*,*,#9822,.T.);
#14344=ORIENTED_EDGE('',*,*,#9773,.F.);
#14345=ORIENTED_EDGE('',*,*,#9824,.T.);
#14346=ORIENTED_EDGE('',*,*,#9827,.F.);
#14347=ORIENTED_EDGE('',*,*,#9828,.T.);
#14348=ORIENTED_EDGE('',*,*,#9826,.T.);
#14349=ORIENTED_EDGE('',*,*,#9828,.F.);
#14350=ORIENTED_EDGE('',*,*,#9829,.F.);
#14351=ORIENTED_EDGE('',*,*,#9827,.T.);
#14352=ORIENTED_EDGE('',*,*,#9830,.F.);
#14353=ORIENTED_EDGE('',*,*,#9831,.T.);
#14354=ORIENTED_EDGE('',*,*,#9829,.T.);
#14355=ORIENTED_EDGE('',*,*,#9831,.F.);
#14356=ORIENTED_EDGE('',*,*,#9832,.F.);
#14357=ORIENTED_EDGE('',*,*,#9833,.T.);
#14358=ORIENTED_EDGE('',*,*,#9830,.T.);
#14359=ORIENTED_EDGE('',*,*,#9833,.F.);
#14360=ORIENTED_EDGE('',*,*,#9832,.T.);
#14361=ORIENTED_EDGE('',*,*,#9820,.T.);
#14362=ORIENTED_EDGE('',*,*,#9778,.F.);
#14363=ORIENTED_EDGE('',*,*,#9823,.T.);
#14364=ORIENTED_EDGE('',*,*,#9782,.T.);
#15946=PLANE('',#18629);
#15947=PLANE('',#18634);
#15948=PLANE('',#18640);
#16796=ADVANCED_FACE('',(#2987),#334,.F.);
#16797=ADVANCED_FACE('',(#2988),#335,.F.);
#16798=ADVANCED_FACE('',(#2989),#336,.F.);
#16799=ADVANCED_FACE('',(#2990),#337,.F.);
#16800=ADVANCED_FACE('',(#2991),#338,.F.);
#16801=ADVANCED_FACE('',(#2992),#339,.F.);
#16802=ADVANCED_FACE('',(#2993),#340,.F.);
#16803=ADVANCED_FACE('',(#2994),#341,.F.);
#16804=ADVANCED_FACE('',(#2995),#342,.F.);
#16805=ADVANCED_FACE('',(#2996),#343,.F.);
#16806=ADVANCED_FACE('',(#2997),#344,.F.);
#16807=ADVANCED_FACE('',(#2998),#345,.F.);
#16808=ADVANCED_FACE('',(#2999),#346,.F.);
#16809=ADVANCED_FACE('',(#3000),#347,.F.);
#16810=ADVANCED_FACE('',(#3001),#348,.F.);
#16811=ADVANCED_FACE('',(#3002),#349,.F.);
#16812=ADVANCED_FACE('',(#3003),#350,.F.);
#16813=ADVANCED_FACE('',(#3004),#351,.F.);
#16814=ADVANCED_FACE('',(#3005),#352,.F.);
#16815=ADVANCED_FACE('',(#3006),#353,.F.);
#16816=ADVANCED_FACE('',(#3007),#354,.F.);
#16817=ADVANCED_FACE('',(#3008),#355,.F.);
#16818=ADVANCED_FACE('',(#3009),#356,.F.);
#16819=ADVANCED_FACE('',(#3010),#357,.F.);
#16820=ADVANCED_FACE('',(#3011),#358,.F.);
#16821=ADVANCED_FACE('',(#3012),#76,.F.);
#16822=ADVANCED_FACE('',(#3013),#77,.F.);
#16823=ADVANCED_FACE('',(#3014,#1462),#15946,.T.);
#16824=ADVANCED_FACE('',(#3015),#359,.F.);
#16825=ADVANCED_FACE('',(#3016),#360,.T.);
#16826=ADVANCED_FACE('',(#3017,#1463),#15947,.T.);
#16827=ADVANCED_FACE('',(#3018),#361,.T.);
#16828=ADVANCED_FACE('',(#3019),#1028,.T.);
#16829=ADVANCED_FACE('',(#3020,#1464),#15948,.T.);
#17074=CLOSED_SHELL('',(#16796,#16797,#16798,#16799,#16800,#16801,#16802,
#16803,#16804,#16805,#16806,#16807,#16808,#16809,#16810,#16811,#16812,#16813,
#16814,#16815,#16816,#16817,#16818,#16819,#16820,#16821,#16822,#16823,#16824,
#16825,#16826,#16827,#16828,#16829));
#18599=AXIS2_PLACEMENT_3D('',#28601,#22475,#22476);
#18600=AXIS2_PLACEMENT_3D('',#28602,#22477,#22478);
#18601=AXIS2_PLACEMENT_3D('',#28633,#22480,#22481);
#18602=AXIS2_PLACEMENT_3D('',#28671,#22482,#22483);
#18603=AXIS2_PLACEMENT_3D('',#28758,#22485,#22486);
#18604=AXIS2_PLACEMENT_3D('',#28848,#22488,#22489);
#18605=AXIS2_PLACEMENT_3D('',#28935,#22491,#22492);
#18606=AXIS2_PLACEMENT_3D('',#29022,#22494,#22495);
#18607=AXIS2_PLACEMENT_3D('',#29112,#22497,#22498);
#18608=AXIS2_PLACEMENT_3D('',#29199,#22500,#22501);
#18609=AXIS2_PLACEMENT_3D('',#29286,#22503,#22504);
#18610=AXIS2_PLACEMENT_3D('',#29376,#22506,#22507);
#18611=AXIS2_PLACEMENT_3D('',#29463,#22509,#22510);
#18612=AXIS2_PLACEMENT_3D('',#29550,#22512,#22513);
#18613=AXIS2_PLACEMENT_3D('',#29563,#22515,#22516);
#18614=AXIS2_PLACEMENT_3D('',#29580,#22517,#22518);
#18615=AXIS2_PLACEMENT_3D('',#29598,#22520,#22521);
#18616=AXIS2_PLACEMENT_3D('',#29613,#22522,#22523);
#18617=AXIS2_PLACEMENT_3D('',#29650,#22525,#22526);
#18618=AXIS2_PLACEMENT_3D('',#29688,#22528,#22529);
#18619=AXIS2_PLACEMENT_3D('',#29725,#22531,#22532);
#18620=AXIS2_PLACEMENT_3D('',#29762,#22534,#22535);
#18621=AXIS2_PLACEMENT_3D('',#29800,#22537,#22538);
#18622=AXIS2_PLACEMENT_3D('',#29837,#22540,#22541);
#18623=AXIS2_PLACEMENT_3D('',#29874,#22543,#22544);
#18624=AXIS2_PLACEMENT_3D('',#29912,#22546,#22547);
#18625=AXIS2_PLACEMENT_3D('',#29949,#22549,#22550);
#18626=AXIS2_PLACEMENT_3D('',#29986,#22552,#22553);
#18627=AXIS2_PLACEMENT_3D('',#29998,#22555,#22556);
#18628=AXIS2_PLACEMENT_3D('',#30006,#22557,#22558);
#18629=AXIS2_PLACEMENT_3D('',#31877,#22559,#22560);
#18630=AXIS2_PLACEMENT_3D('',#31879,#22561,#22562);
#18631=AXIS2_PLACEMENT_3D('',#31880,#22563,#22564);
#18632=AXIS2_PLACEMENT_3D('',#31881,#22565,#22566);
#18633=AXIS2_PLACEMENT_3D('',#31883,#22567,#22568);
#18634=AXIS2_PLACEMENT_3D('',#31885,#22570,#22571);
#18635=AXIS2_PLACEMENT_3D('',#31887,#22572,#22573);
#18636=AXIS2_PLACEMENT_3D('',#31888,#22574,#22575);
#18637=AXIS2_PLACEMENT_3D('',#31890,#22576,#22577);
#18638=AXIS2_PLACEMENT_3D('',#31892,#22579,#22580);
#18639=AXIS2_PLACEMENT_3D('',#31894,#22581,#22582);
#18640=AXIS2_PLACEMENT_3D('',#31896,#22584,#22585);
#22475=DIRECTION('axis',(0.,0.,1.));
#22476=DIRECTION('refdir',(1.,0.,0.));
#22477=DIRECTION('center_axis',(1.,0.,0.));
#22478=DIRECTION('ref_axis',(0.,0.935047775444299,0.354521730838417));
#22479=DIRECTION('',(-1.,0.,0.));
#22480=DIRECTION('center_axis',(-1.,0.,0.));
#22481=DIRECTION('ref_axis',(0.,1.,0.));
#22482=DIRECTION('center_axis',(1.,0.,0.));
#22483=DIRECTION('ref_axis',(0.,1.,0.));
#22484=DIRECTION('',(-1.,0.,0.));
#22485=DIRECTION('center_axis',(1.,0.,0.));
#22486=DIRECTION('ref_axis',(0.,1.,0.));
#22487=DIRECTION('',(-1.,0.,0.));
#22488=DIRECTION('center_axis',(1.,0.,0.));
#22489=DIRECTION('ref_axis',(0.,1.,0.));
#22490=DIRECTION('',(-1.,0.,0.));
#22491=DIRECTION('center_axis',(1.,0.,0.));
#22492=DIRECTION('ref_axis',(0.,1.,0.));
#22493=DIRECTION('',(-1.,0.,0.));
#22494=DIRECTION('center_axis',(1.,0.,0.));
#22495=DIRECTION('ref_axis',(0.,1.,0.));
#22496=DIRECTION('',(-1.,0.,0.));
#22497=DIRECTION('center_axis',(1.,0.,0.));
#22498=DIRECTION('ref_axis',(0.,1.,0.));
#22499=DIRECTION('',(-1.,0.,0.));
#22500=DIRECTION('center_axis',(1.,0.,0.));
#22501=DIRECTION('ref_axis',(0.,1.,0.));
#22502=DIRECTION('',(-1.,0.,0.));
#22503=DIRECTION('center_axis',(1.,0.,0.));
#22504=DIRECTION('ref_axis',(0.,1.,0.));
#22505=DIRECTION('',(-1.,0.,0.));
#22506=DIRECTION('center_axis',(1.,0.,0.));
#22507=DIRECTION('ref_axis',(0.,1.,0.));
#22508=DIRECTION('',(-1.,0.,0.));
#22509=DIRECTION('center_axis',(1.,0.,0.));
#22510=DIRECTION('ref_axis',(0.,1.,0.));
#22511=DIRECTION('',(-1.,0.,0.));
#22512=DIRECTION('center_axis',(1.,0.,0.));
#22513=DIRECTION('ref_axis',(0.,-0.354512791606023,-0.935051164689775));
#22514=DIRECTION('',(-1.,0.,0.));
#22515=DIRECTION('center_axis',(1.,0.,0.));
#22516=DIRECTION('ref_axis',(0.,1.,0.));
#22517=DIRECTION('center_axis',(1.,0.,0.));
#22518=DIRECTION('ref_axis',(0.,0.793330745045896,-0.608790874574286));
#22519=DIRECTION('',(1.,1.22464679914735E-16,5.71605565684554E-30));
#22520=DIRECTION('center_axis',(-1.,0.,0.));
#22521=DIRECTION('ref_axis',(0.,1.,4.65526718641507E-14));
#22522=DIRECTION('center_axis',(1.,0.,0.));
#22523=DIRECTION('ref_axis',(0.,1.,4.65526718641507E-14));
#22524=DIRECTION('',(1.,1.22464679914735E-16,5.71605565684554E-30));
#22525=DIRECTION('center_axis',(1.,0.,0.));
#22526=DIRECTION('ref_axis',(0.,1.,4.65526718641507E-14));
#22527=DIRECTION('',(1.,1.22464679914735E-16,5.71605565684554E-30));
#22528=DIRECTION('center_axis',(1.,0.,0.));
#22529=DIRECTION('ref_axis',(0.,1.,4.65526718641507E-14));
#22530=DIRECTION('',(1.,1.22464679914735E-16,5.71605565684554E-30));
#22531=DIRECTION('center_axis',(1.,0.,0.));
#22532=DIRECTION('ref_axis',(0.,1.,4.65526718641507E-14));
#22533=DIRECTION('',(1.,1.22464679914735E-16,5.71605565684554E-30));
#22534=DIRECTION('center_axis',(1.,0.,0.));
#22535=DIRECTION('ref_axis',(0.,1.,4.65526718641507E-14));
#22536=DIRECTION('',(1.,1.22464679914735E-16,5.71605565684554E-30));
#22537=DIRECTION('center_axis',(1.,0.,0.));
#22538=DIRECTION('ref_axis',(0.,1.,4.65526718641507E-14));
#22539=DIRECTION('',(1.,1.22464679914735E-16,5.71605565684554E-30));
#22540=DIRECTION('center_axis',(1.,0.,0.));
#22541=DIRECTION('ref_axis',(0.,1.,4.65526718641507E-14));
#22542=DIRECTION('',(1.,1.22464679914735E-16,5.71605565684554E-30));
#22543=DIRECTION('center_axis',(1.,0.,0.));
#22544=DIRECTION('ref_axis',(0.,1.,4.65526718641507E-14));
#22545=DIRECTION('',(1.,1.22464679914735E-16,5.71605565684554E-30));
#22546=DIRECTION('center_axis',(1.,0.,0.));
#22547=DIRECTION('ref_axis',(0.,1.,4.65526718641507E-14));
#22548=DIRECTION('',(1.,1.22464679914735E-16,5.71605565684554E-30));
#22549=DIRECTION('center_axis',(1.,0.,0.));
#22550=DIRECTION('ref_axis',(0.,1.,4.65526718641507E-14));
#22551=DIRECTION('',(1.,1.22464679914735E-16,5.71605565684554E-30));
#22552=DIRECTION('center_axis',(1.,0.,0.));
#22553=DIRECTION('ref_axis',(0.,-0.60879845580878,0.793324927255437));
#22554=DIRECTION('',(1.,1.22464679914735E-16,5.71605565684554E-30));
#22555=DIRECTION('center_axis',(1.,0.,0.));
#22556=DIRECTION('ref_axis',(0.,1.,4.65526718641507E-14));
#22557=DIRECTION('center_axis',(1.,0.,0.));
#22558=DIRECTION('ref_axis',(0.,1.,4.65526718641507E-14));
#22559=DIRECTION('center_axis',(-1.,0.,0.));
#22560=DIRECTION('ref_axis',(0.,0.,1.));
#22561=DIRECTION('center_axis',(1.,0.,0.));
#22562=DIRECTION('ref_axis',(0.,0.,-1.));
#22563=DIRECTION('center_axis',(1.,0.,0.));
#22564=DIRECTION('ref_axis',(0.,1.,0.));
#22565=DIRECTION('center_axis',(1.,0.,0.));
#22566=DIRECTION('ref_axis',(0.,1.,0.));
#22567=DIRECTION('center_axis',(1.,0.,0.));
#22568=DIRECTION('ref_axis',(0.,0.,-1.));
#22569=DIRECTION('',(-1.,0.,0.));
#22570=DIRECTION('center_axis',(-1.,0.,0.));
#22571=DIRECTION('ref_axis',(0.,0.,1.));
#22572=DIRECTION('center_axis',(1.,0.,0.));
#22573=DIRECTION('ref_axis',(0.,0.,-1.));
#22574=DIRECTION('center_axis',(1.,0.,0.));
#22575=DIRECTION('ref_axis',(0.,1.,0.));
#22576=DIRECTION('center_axis',(1.,0.,0.));
#22577=DIRECTION('ref_axis',(0.,0.,-1.));
#22578=DIRECTION('',(-1.,0.,0.));
#22579=DIRECTION('center_axis',(-1.,0.,0.));
#22580=DIRECTION('ref_axis',(0.,1.,0.));
#22581=DIRECTION('center_axis',(1.,0.,0.));
#22582=DIRECTION('ref_axis',(0.,0.,-1.));
#22583=DIRECTION('',(-0.707106781186547,-0.707106781186548,-8.65956056235493E-17));
#22584=DIRECTION('center_axis',(1.,0.,0.));
#22585=DIRECTION('ref_axis',(0.,0.,-1.));
#28601=CARTESIAN_POINT('',(0.,0.,0.));
#28602=CARTESIAN_POINT('Origin',(-3.5,0.,0.));
#28603=CARTESIAN_POINT('',(-7.33651593783807,-9.64123956416204,0.000230242740474756));
#28604=CARTESIAN_POINT('',(-7.53848406216193,-9.64164981768271,-0.000239867588180398));
#28605=CARTESIAN_POINT('',(-3.5,-9.64155,-1.18074933463192E-15));
#28606=CARTESIAN_POINT('',(-8.,7.21801009705396,-6.39216838336781));
#28607=CARTESIAN_POINT('Ctrl Pts',(-7.53848406216193,-9.64164981768271,
-0.000239867588180398));
#28608=CARTESIAN_POINT('Ctrl Pts',(-7.55407606170334,-9.64036790708282,
1.25910592241467));
#28609=CARTESIAN_POINT('Ctrl Pts',(-7.56966806124475,-9.39229948530074,
2.51894068414412));
#28610=CARTESIAN_POINT('Ctrl Pts',(-7.58526006078616,-8.91143640847641,
3.6825791927546));
#28611=CARTESIAN_POINT('Ctrl Pts',(-7.6050095817011,-8.30235382302952,5.1564955433938));
#28612=CARTESIAN_POINT('Ctrl Pts',(-7.62475910261605,-7.31977820211336,
6.47607574498501));
#28613=CARTESIAN_POINT('Ctrl Pts',(-7.64450862353099,-6.08227773070946,
7.48205342360144));
#28614=CARTESIAN_POINT('Ctrl Pts',(-7.66425814444594,-4.84477725930556,
8.48803110221788));
#28615=CARTESIAN_POINT('Ctrl Pts',(-7.68400766536088,-3.35235193741391,
9.18040625785953));
#28616=CARTESIAN_POINT('Ctrl Pts',(-7.70375718627582,-1.78511818710048,
9.47566722361494));
#28617=CARTESIAN_POINT('Ctrl Pts',(-7.72350670719077,-0.21788443678705,
9.77092818937035));
#28618=CARTESIAN_POINT('Ctrl Pts',(-7.74325622810571,1.42415774194816,9.66907496523952));
#28619=CARTESIAN_POINT('Ctrl Pts',(-7.76300574902066,2.94287634303685,9.18231633088148));
#28620=CARTESIAN_POINT('Ctrl Pts',(-7.78275526993561,4.46159494412553,8.69555769652344));
#28621=CARTESIAN_POINT('Ctrl Pts',(-7.80250479085055,5.8569899675677,7.82389365193819));
#28622=CARTESIAN_POINT('Ctrl Pts',(-7.8222543117655,6.96061672529205,6.67267543875423));
#28623=CARTESIAN_POINT('Ctrl Pts',(-7.84200383268044,8.0642434830164,5.52145722557028));
#28624=CARTESIAN_POINT('Ctrl Pts',(-7.86175335359539,8.87610197502294,4.09068484378763));
#28625=CARTESIAN_POINT('Ctrl Pts',(-7.88150287451033,9.29832265436953,2.55270136385008));
#28626=CARTESIAN_POINT('Ctrl Pts',(-7.90125239542527,9.72054333371612,1.01471788391252));
#28627=CARTESIAN_POINT('Ctrl Pts',(-7.92100191634022,9.75312620040277,-0.630476694179928));
#28628=CARTESIAN_POINT('Ctrl Pts',(-7.94075143725517,9.39189406895472,-2.18363754482683));
#28629=CARTESIAN_POINT('Ctrl Pts',(-7.96050095817011,9.03066193750668,-3.73679839547375));
#28630=CARTESIAN_POINT('Ctrl Pts',(-7.98025047908506,8.27561480792393,-5.19792551867511));
#28631=CARTESIAN_POINT('Ctrl Pts',(-8.,7.21801009705396,-6.39216838336781));
#28632=CARTESIAN_POINT('',(-8.,-7.21857424983126,-6.39248700007983));
#28633=CARTESIAN_POINT('Origin',(-8.,0.,0.));
#28634=CARTESIAN_POINT('Ctrl Pts',(-8.,-7.21857424983126,-6.39248700007983));
#28635=CARTESIAN_POINT('Ctrl Pts',(-7.98217765815669,-6.26356488414857,
-7.46927134726881));
#28636=CARTESIAN_POINT('Ctrl Pts',(-7.96435531631337,-5.06448313044863,
-8.33050691837291));
#28637=CARTESIAN_POINT('Ctrl Pts',(-7.94653297447006,-3.73783082080585,
-8.88839335033359));
#28638=CARTESIAN_POINT('Ctrl Pts',(-7.92678345355512,-2.26772393101004,
-9.50660558377841));
#28639=CARTESIAN_POINT('Ctrl Pts',(-7.90703393264017,-0.640965728279816,
-9.75231774796247));
#28640=CARTESIAN_POINT('Ctrl Pts',(-7.88728441172523,0.946142179189394,
-9.59583455621896));
#28641=CARTESIAN_POINT('Ctrl Pts',(-7.86753489081029,2.53325008665859,-9.43935136447544));
#28642=CARTESIAN_POINT('Ctrl Pts',(-7.84778536989534,4.08070769886678,-8.88067281680435));
#28643=CARTESIAN_POINT('Ctrl Pts',(-7.82803584898039,5.40176465239776,-7.98724149155587));
#28644=CARTESIAN_POINT('Ctrl Pts',(-7.80828632806545,6.72282160592874,-7.09381016630739));
#28645=CARTESIAN_POINT('Ctrl Pts',(-7.7885368071505,7.81747790078251,-5.86562606348152));
#28646=CARTESIAN_POINT('Ctrl Pts',(-7.76878728623556,8.55363593826125,-4.4508923313193));
#28647=CARTESIAN_POINT('Ctrl Pts',(-7.74903776532061,9.28979397573999,-3.03615859915706));
#28648=CARTESIAN_POINT('Ctrl Pts',(-7.72928824440567,9.66745375584369,-1.43487523765846));
#28649=CARTESIAN_POINT('Ctrl Pts',(-7.70953872349072,9.64103836683124,0.159712143192118));
#28650=CARTESIAN_POINT('Ctrl Pts',(-7.68978920257578,9.61462297781878,1.75429952404268));
#28651=CARTESIAN_POINT('Ctrl Pts',(-7.67003968166083,9.18413241969018,3.34219092424522));
#28652=CARTESIAN_POINT('Ctrl Pts',(-7.65029016074589,8.40151829426746,4.73176596758706));
#28653=CARTESIAN_POINT('Ctrl Pts',(-7.63054063983094,7.61890416884475,6.1213410109289));
#28654=CARTESIAN_POINT('Ctrl Pts',(-7.61079111891599,6.48416647612792,7.31259969741003));
#28655=CARTESIAN_POINT('Ctrl Pts',(-7.59104159800105,5.13424258452846,8.16178175236003));
#28656=CARTESIAN_POINT('Ctrl Pts',(-7.57129207708611,3.78431869292901,9.01096380731002));
#28657=CARTESIAN_POINT('Ctrl Pts',(-7.55154255617117,2.21920860244693,9.51806923072888));
#28658=CARTESIAN_POINT('Ctrl Pts',(-7.53179303525622,0.627786835584183,
9.62190241167914));
#28659=CARTESIAN_POINT('Ctrl Pts',(-7.51204351434128,-0.963634931278574,
9.7257355926294));
#28660=CARTESIAN_POINT('Ctrl Pts',(-7.49229399342633,-2.581368374522,9.42629653111106));
#28661=CARTESIAN_POINT('Ctrl Pts',(-7.47254447251138,-4.03018885195262,
8.75972048847779));
#28662=CARTESIAN_POINT('Ctrl Pts',(-7.45279495159643,-5.47900932938324,
8.09314444584453));
#28663=CARTESIAN_POINT('Ctrl Pts',(-7.43304543068149,-6.75891684100106,
7.05943142209633));
#28664=CARTESIAN_POINT('Ctrl Pts',(-7.41329590976655,-7.71545470147883,
5.78332801562085));
#28665=CARTESIAN_POINT('Ctrl Pts',(-7.3935463888516,-8.67199256195661,4.50722460914537));
#28666=CARTESIAN_POINT('Ctrl Pts',(-7.37379686793666,-9.30516077129434,
2.9887308199426));
#28667=CARTESIAN_POINT('Ctrl Pts',(-7.35404734702171,-9.53854991728423,
1.41109525810262));
#28668=CARTESIAN_POINT('Ctrl Pts',(-7.3482035439605,-9.60760881808813,0.944279300112268));
#28669=CARTESIAN_POINT('Ctrl Pts',(-7.34235974089929,-9.64166529987996,
0.472285219261674));
#28670=CARTESIAN_POINT('Ctrl Pts',(-7.33651593783807,-9.64123956416204,
0.000230242740474756));
#28671=CARTESIAN_POINT('Origin',(-3.5,0.,0.));
#28672=CARTESIAN_POINT('',(-6.58651593783807,-9.64231270617946,-7.42785913304498E-5));
#28673=CARTESIAN_POINT('',(-6.78848406216194,-9.64077611273789,7.46528660069967E-5));
#28674=CARTESIAN_POINT('',(-3.5,-9.64155,-1.18074933463192E-15));
#28675=CARTESIAN_POINT('Ctrl Pts',(-6.78848406216194,-9.64077611273789,
7.46528660069967E-5));
#28676=CARTESIAN_POINT('Ctrl Pts',(-6.79733228980906,-9.64097151845064,
0.714921728157376));
#28677=CARTESIAN_POINT('Ctrl Pts',(-6.80618051745618,-9.56250642288335,
1.42972656374862));
#28678=CARTESIAN_POINT('Ctrl Pts',(-6.8150287451033,-9.40492023678117,2.12664053828175));
#28679=CARTESIAN_POINT('Ctrl Pts',(-6.83477826601825,-9.05318293949953,
3.68217433158735));
#28680=CARTESIAN_POINT('Ctrl Pts',(-6.85452778693319,-8.30726724506208,
5.14857650539751));
#28681=CARTESIAN_POINT('Ctrl Pts',(-6.87427730784814,-7.2571887358938,6.34888464751866));
#28682=CARTESIAN_POINT('Ctrl Pts',(-6.89402682876308,-6.20711022672555,
7.5491927896398));
#28683=CARTESIAN_POINT('Ctrl Pts',(-6.91377634967803,-4.85286890282648,
8.48340690007195));
#28684=CARTESIAN_POINT('Ctrl Pts',(-6.93352587059297,-3.35789183596898,
9.0387879216256));
#28685=CARTESIAN_POINT('Ctrl Pts',(-6.95327539150792,-1.86291476911148,
9.59416894317926));
#28686=CARTESIAN_POINT('Ctrl Pts',(-6.97302491242286,-0.227201959295531,
9.77071687585441));
#28687=CARTESIAN_POINT('Ctrl Pts',(-6.99277443333781,1.35185211055659,9.54712629195822));
#28688=CARTESIAN_POINT('Ctrl Pts',(-7.01252395425275,2.93090618040872,9.32353570806203));
#28689=CARTESIAN_POINT('Ctrl Pts',(-7.0322734751677,4.45330151029702,8.69980660759449));
#28690=CARTESIAN_POINT('Ctrl Pts',(-7.05202299608264,5.73531855391222,7.75120931257361));
#28691=CARTESIAN_POINT('Ctrl Pts',(-7.07177251699759,7.01733559752742,6.80261201755272));
#28692=CARTESIAN_POINT('Ctrl Pts',(-7.09152203791253,8.05897435486951,5.52914652797849));
#28693=CARTESIAN_POINT('Ctrl Pts',(-7.11127155882748,8.73453197137747,4.08449211495003));
#28694=CARTESIAN_POINT('Ctrl Pts',(-7.13102107974242,9.41008958788543,2.63983770192156));
#28695=CARTESIAN_POINT('Ctrl Pts',(-7.15077060065737,9.71956606355925,1.02399436543886));
#28696=CARTESIAN_POINT('Ctrl Pts',(-7.17052012157232,9.6256144463609,-0.568041338486824));
#28697=CARTESIAN_POINT('Ctrl Pts',(-7.19026964248726,9.53166282916255,-2.16007704241249));
#28698=CARTESIAN_POINT('Ctrl Pts',(-7.21001916340221,9.03428311909205,-3.72830511378114));
#28699=CARTESIAN_POINT('Ctrl Pts',(-7.22976868431715,8.19349801251508,-5.08347477399469));
#28700=CARTESIAN_POINT('Ctrl Pts',(-7.24951820523209,7.35271290593811,-6.43864443420824));
#28701=CARTESIAN_POINT('Ctrl Pts',(-7.26926772614704,6.16852240285469,-7.58075568326669));
#28702=CARTESIAN_POINT('Ctrl Pts',(-7.28901724706198,4.78383232783281,-8.37198129730586));
#28703=CARTESIAN_POINT('Ctrl Pts',(-7.30876676797693,3.39914225281091,-9.16320691134503));
#28704=CARTESIAN_POINT('Ctrl Pts',(-7.32851628889188,1.81395260585056,-9.60354689036491));
#28705=CARTESIAN_POINT('Ctrl Pts',(-7.34826580980682,0.219560570984832,
-9.63986108179457));
#28706=CARTESIAN_POINT('Ctrl Pts',(-7.36801533072177,-1.3748314638809,-9.67617527322422));
#28707=CARTESIAN_POINT('Ctrl Pts',(-7.38776485163671,-2.97842588665202,
-9.30846367706364));
#28708=CARTESIAN_POINT('Ctrl Pts',(-7.40751437255165,-4.39770369511272,
-8.58110256845882));
#28709=CARTESIAN_POINT('Ctrl Pts',(-7.4272638934666,-5.81698150357342,-7.85374145985401));
#28710=CARTESIAN_POINT('Ctrl Pts',(-7.44701341438155,-7.05194269772371,
-6.76673083880497));
#28711=CARTESIAN_POINT('Ctrl Pts',(-7.46676293529649,-7.95355566179962,
-5.45124585153094));
#28712=CARTESIAN_POINT('Ctrl Pts',(-7.48651245621144,-8.85516862587553,
-4.13576086425692));
#28713=CARTESIAN_POINT('Ctrl Pts',(-7.50626197712638,-9.42343335987706,
-2.59180151075793));
#28714=CARTESIAN_POINT('Ctrl Pts',(-7.52601149804132,-9.58977095188901,
-1.00569558416484));
#28715=CARTESIAN_POINT('Ctrl Pts',(-7.53016901941486,-9.62478709719151,
-0.671800432028954));
#28716=CARTESIAN_POINT('Ctrl Pts',(-7.5343265407884,-9.64199163213081,-0.336037532583489));
#28717=CARTESIAN_POINT('Ctrl Pts',(-7.53848406216193,-9.64164981768271,
-0.000239867588180398));
#28718=CARTESIAN_POINT('Ctrl Pts',(-7.33651593783807,-9.64123956416204,
0.000230242740474756));
#28719=CARTESIAN_POINT('Ctrl Pts',(-7.32261021998434,-9.64022649772028,
-1.12305595396952));
#28720=CARTESIAN_POINT('Ctrl Pts',(-7.30870450213061,-9.44396350863798,
-2.24668696246466));
#28721=CARTESIAN_POINT('Ctrl Pts',(-7.29479878427688,-9.05945974325286,
-3.30171374270337));
#28722=CARTESIAN_POINT('Ctrl Pts',(-7.27504926336193,-8.51337034058954,
-4.80010984719222));
#28723=CARTESIAN_POINT('Ctrl Pts',(-7.25529974244699,-7.58758145262085,
-6.16012472169274));
#28724=CARTESIAN_POINT('Ctrl Pts',(-7.23555022153204,-6.39381539850043,
-7.21763458266072));
#28725=CARTESIAN_POINT('Ctrl Pts',(-7.2158007006171,-5.20004934438002,-8.2751444436287));
#28726=CARTESIAN_POINT('Ctrl Pts',(-7.19605117970216,-3.73830612410787,
-9.03014929106414));
#28727=CARTESIAN_POINT('Ctrl Pts',(-7.17630165878721,-2.1849859165843,-9.39153666737156));
#28728=CARTESIAN_POINT('Ctrl Pts',(-7.15655213787226,-0.63166570906074,
-9.75292404367897));
#28729=CARTESIAN_POINT('Ctrl Pts',(-7.13680261695732,1.01323148571424,-9.72069394885837));
#28730=CARTESIAN_POINT('Ctrl Pts',(-7.11705309604237,2.55120283470161,-9.29873585321303));
#28731=CARTESIAN_POINT('Ctrl Pts',(-7.09730357512743,4.08917418368899,-8.8767777575677));
#28732=CARTESIAN_POINT('Ctrl Pts',(-7.07755405421249,5.52021968688874,-8.06509166109762));
#28733=CARTESIAN_POINT('Ctrl Pts',(-7.05780453329754,6.67164369979784,-6.96163017820614));
#28734=CARTESIAN_POINT('Ctrl Pts',(-7.03805501238259,7.82306771270693,-5.85816869531467));
#28735=CARTESIAN_POINT('Ctrl Pts',(-7.01830549146764,8.69487023532537,-4.46293182600177));
#28736=CARTESIAN_POINT('Ctrl Pts',(-6.9985559705527,9.18184392088289,-2.94429390550503));
#28737=CARTESIAN_POINT('Ctrl Pts',(-6.97880644963775,9.6688176064404,-1.42565598500829));
#28738=CARTESIAN_POINT('Ctrl Pts',(-6.95905692872282,9.77096245493699,0.216382986672299));
#28739=CARTESIAN_POINT('Ctrl Pts',(-6.93930740780787,9.47595183520748,1.78366510454321));
#28740=CARTESIAN_POINT('Ctrl Pts',(-6.91955788689293,9.18094121547797,3.35094722241412));
#28741=CARTESIAN_POINT('Ctrl Pts',(-6.89980836597798,8.48877512752234,4.84347248647533));
#28742=CARTESIAN_POINT('Ctrl Pts',(-6.88005884506304,7.48298275961571,6.08112599854471));
#28743=CARTESIAN_POINT('Ctrl Pts',(-6.86030932414809,6.47719039170906,7.3187795106141));
#28744=CARTESIAN_POINT('Ctrl Pts',(-6.84055980323314,5.15777174385139,8.30156127069164));
#28745=CARTESIAN_POINT('Ctrl Pts',(-6.8208102823182,3.68395156116386,8.91087118545994));
#28746=CARTESIAN_POINT('Ctrl Pts',(-6.80106076140325,2.21013137847635,9.52018110022824));
#28747=CARTESIAN_POINT('Ctrl Pts',(-6.78131124048831,0.58190966095899,9.7560191696873));
#28748=CARTESIAN_POINT('Ctrl Pts',(-6.76156171957337,-1.0042231232646,9.58992493759571));
#28749=CARTESIAN_POINT('Ctrl Pts',(-6.74181219865842,-2.59035590748818,
9.42383070550413));
#28750=CARTESIAN_POINT('Ctrl Pts',(-6.72206267774348,-4.13439975841799,
8.85580417186189));
#28751=CARTESIAN_POINT('Ctrl Pts',(-6.70231315682853,-5.45002262070945,
7.95439361757151));
#28752=CARTESIAN_POINT('Ctrl Pts',(-6.68256363591358,-6.76564548300091,
7.05298306328113));
#28753=CARTESIAN_POINT('Ctrl Pts',(-6.66281411499864,-7.85284735665405,
5.81818848834261));
#28754=CARTESIAN_POINT('Ctrl Pts',(-6.64306459408369,-8.58042694222024,
4.39902237762939));
#28755=CARTESIAN_POINT('Ctrl Pts',(-6.62421504200182,-9.27485134628063,
3.04452645684594));
#28756=CARTESIAN_POINT('Ctrl Pts',(-6.60536548991995,-9.64168205182771,
1.52207945153344));
#28757=CARTESIAN_POINT('Ctrl Pts',(-6.58651593783807,-9.64231270617946,
-7.42785913304498E-5));
#28758=CARTESIAN_POINT('Origin',(-3.5,0.,0.));
#28759=CARTESIAN_POINT('',(-5.83651593783807,-9.6409035792506,-0.000152919944957977));
#28760=CARTESIAN_POINT('',(-6.03848406216193,-9.6421289025524,0.00016016297285322));
#28761=CARTESIAN_POINT('',(-3.5,-9.64155,-1.18074933463192E-15));
#28762=CARTESIAN_POINT('Ctrl Pts',(-6.03848406216193,-9.6421289025524,0.00016016297285322));
#28763=CARTESIAN_POINT('Ctrl Pts',(-6.04058851791477,-9.6422628445658,0.170110221396648));
#28764=CARTESIAN_POINT('Ctrl Pts',(-6.04269297366761,-9.63786113934538,
0.340053343096354));
#28765=CARTESIAN_POINT('Ctrl Pts',(-6.04479742942045,-9.62887717318408,
0.509753879367992));
#28766=CARTESIAN_POINT('Ctrl Pts',(-6.0645469503354,-9.54456605029038,2.10232919764383));
#28767=CARTESIAN_POINT('Ctrl Pts',(-6.08429647125035,-9.05669006237452,
3.67353974494806));
#28768=CARTESIAN_POINT('Ctrl Pts',(-6.10404599216529,-8.22412508625499,
5.03377504457948));
#28769=CARTESIAN_POINT('Ctrl Pts',(-6.12379551308023,-7.39156011013546,
6.3940103442109));
#28770=CARTESIAN_POINT('Ctrl Pts',(-6.14354503399518,-6.21430614581225,
7.54327039616953));
#28771=CARTESIAN_POINT('Ctrl Pts',(-6.16329455491012,-4.83443179494827,
8.34286484690855));
#28772=CARTESIAN_POINT('Ctrl Pts',(-6.18304407582506,-3.45455744408426,
9.14245929764759));
#28773=CARTESIAN_POINT('Ctrl Pts',(-6.20279359674001,-1.87206270667947,
9.59238814716702));
#28774=CARTESIAN_POINT('Ctrl Pts',(-6.22254311765496,-0.277919812425482,
9.63835490172843));
#28775=CARTESIAN_POINT('Ctrl Pts',(-6.2422926385699,1.3162230818285,9.68432165628985));
#28776=CARTESIAN_POINT('Ctrl Pts',(-6.26204215948485,2.92201413293167,9.32632631589325));
#28777=CARTESIAN_POINT('Ctrl Pts',(-6.28179168039979,4.34566975967897,8.6075710263458));
#28778=CARTESIAN_POINT('Ctrl Pts',(-6.30154120131473,5.76932538642627,7.88881573679835));
#28779=CARTESIAN_POINT('Ctrl Pts',(-6.32129072222968,7.01084558881768,6.80930049810006));
#28780=CARTESIAN_POINT('Ctrl Pts',(-6.34104024314462,7.92040624696886,5.49929900230839));
#28781=CARTESIAN_POINT('Ctrl Pts',(-6.36078976405957,8.82996690512002,4.18929750651673));
#28782=CARTESIAN_POINT('Ctrl Pts',(-6.38053928497452,9.40756801903096,2.6488097536317));
#28783=CARTESIAN_POINT('Ctrl Pts',(-6.40028880588946,9.5835058671029,1.06373865635419));
#28784=CARTESIAN_POINT('Ctrl Pts',(-6.42003832680441,9.75944371517485,-0.521332440923332));
#28785=CARTESIAN_POINT('Ctrl Pts',(-6.43978784771935,9.53371829740781,-2.15098688259333));
#28786=CARTESIAN_POINT('Ctrl Pts',(-6.45953736863429,8.93356969576332,-3.62856130230734));
#28787=CARTESIAN_POINT('Ctrl Pts',(-6.47928688954924,8.33342109411885,-5.10613572202132));
#28788=CARTESIAN_POINT('Ctrl Pts',(-6.49903641046419,7.35884930859695,-6.43163011977932));
#28789=CARTESIAN_POINT('Ctrl Pts',(-6.51878593137913,6.12746366985518,-7.44508654138933));
#28790=CARTESIAN_POINT('Ctrl Pts',(-6.53853545229408,4.89607803111339,-8.45854296299935));
#28791=CARTESIAN_POINT('Ctrl Pts',(-6.55828497320902,3.40787853915171,-9.15996140846138));
#28792=CARTESIAN_POINT('Ctrl Pts',(-6.57803449412397,1.84245806626817,-9.4646961339002));
#28793=CARTESIAN_POINT('Ctrl Pts',(-6.59778401503891,0.277037593384629,
-9.76943085933902));
#28794=CARTESIAN_POINT('Ctrl Pts',(-6.61753353595386,-1.36560386042078,
-9.67748186475465));
#28795=CARTESIAN_POINT('Ctrl Pts',(-6.6372830568688,-2.88723568278026,-9.19994536652855));
#28796=CARTESIAN_POINT('Ctrl Pts',(-6.65703257778374,-4.40886750513973,
-8.72240886830246));
#28797=CARTESIAN_POINT('Ctrl Pts',(-6.67678209869869,-5.80948969605326,
-7.85928486643466));
#28798=CARTESIAN_POINT('Ctrl Pts',(-6.69653161961364,-6.92007803273464,
-6.7147334015106));
#28799=CARTESIAN_POINT('Ctrl Pts',(-6.71628114052858,-8.03066636941602,
-5.57018193658653));
#28800=CARTESIAN_POINT('Ctrl Pts',(-6.73603066144353,-8.85122085186524,
-4.14420300860619));
#28801=CARTESIAN_POINT('Ctrl Pts',(-6.75578018235847,-9.28271864302694,
-2.6088808382155));
#28802=CARTESIAN_POINT('Ctrl Pts',(-6.7666814756263,-9.52089576064561,-1.7614173826664));
#28803=CARTESIAN_POINT('Ctrl Pts',(-6.77758276889412,-9.64053536678673,
-0.880639307056883));
#28804=CARTESIAN_POINT('Ctrl Pts',(-6.78848406216194,-9.64077611273789,
7.46528660069967E-5));
#28805=CARTESIAN_POINT('Ctrl Pts',(-6.58651593783807,-9.64231270617946,
-7.42785913304498E-5));
#28806=CARTESIAN_POINT('Ctrl Pts',(-6.585615969005,-9.64234281667007,-0.0727492636680994));
#28807=CARTESIAN_POINT('Ctrl Pts',(-6.58471600017193,-9.64153814863087,
-0.145423580203645));
#28808=CARTESIAN_POINT('Ctrl Pts',(-6.58381603133886,-9.63989450023572,
-0.218078916870951));
#28809=CARTESIAN_POINT('Ctrl Pts',(-6.56406651042392,-9.60382517520572,
-1.81247645417013));
#28810=CARTESIAN_POINT('Ctrl Pts',(-6.54431698950897,-9.16372922766646,
-3.39773388228055));
#28811=CARTESIAN_POINT('Ctrl Pts',(-6.52456746859402,-8.37271653684779,
-4.78254557565492));
#28812=CARTESIAN_POINT('Ctrl Pts',(-6.50481794767908,-7.58170384602911,
-6.16735726902929));
#28813=CARTESIAN_POINT('Ctrl Pts',(-6.48506842676413,-6.43977441193101,
-7.3517232276676));
#28814=CARTESIAN_POINT('Ctrl Pts',(-6.46531890584919,-5.08473394412332,
-8.19271658896709));
#28815=CARTESIAN_POINT('Ctrl Pts',(-6.44556938493425,-3.72969347631562,
-9.03370995026658));
#28816=CARTESIAN_POINT('Ctrl Pts',(-6.4258198640193,-2.16154197479832,-9.53133071422725));
#28817=CARTESIAN_POINT('Ctrl Pts',(-6.40607034310436,-0.569520756880948,
-9.6255270243824));
#28818=CARTESIAN_POINT('Ctrl Pts',(-6.38632082218941,1.02250046103641,-9.71972333453754));
#28819=CARTESIAN_POINT('Ctrl Pts',(-6.36657130127447,2.63839139535383,-9.41049519088718));
#28820=CARTESIAN_POINT('Ctrl Pts',(-6.34682178035952,4.08314963161027,-8.73515961362618));
#28821=CARTESIAN_POINT('Ctrl Pts',(-6.32707225944458,5.52790786786671,-8.05982403636518));
#28822=CARTESIAN_POINT('Ctrl Pts',(-6.30732273852963,6.80153340606216,-7.01838102549355));
#28823=CARTESIAN_POINT('Ctrl Pts',(-6.28757321761468,7.75032772001901,-5.73650979446092));
#28824=CARTESIAN_POINT('Ctrl Pts',(-6.26782369669974,8.69912203397587,-4.45463856342828));
#28825=CARTESIAN_POINT('Ctrl Pts',(-6.2480741757848,9.32308512369412,-2.93233911223461));
#28826=CARTESIAN_POINT('Ctrl Pts',(-6.22832465486985,9.54691839912312,-1.35331942649404));
#28827=CARTESIAN_POINT('Ctrl Pts',(-6.20857513395491,9.77075167455211,0.225700259246526));
#28828=CARTESIAN_POINT('Ctrl Pts',(-6.18882561303996,9.59445513569186,1.86144017953401));
#28829=CARTESIAN_POINT('Ctrl Pts',(-6.16907609212501,9.03930388843518,3.35650258485865));
#28830=CARTESIAN_POINT('Ctrl Pts',(-6.14932657121007,8.48415264117849,4.8515649901833));
#28831=CARTESIAN_POINT('Ctrl Pts',(-6.12957705029513,7.55014668552537,6.2059498805451));
#28832=CARTESIAN_POINT('Ctrl Pts',(-6.10982752938018,6.34999995074282,7.25621285624999));
#28833=CARTESIAN_POINT('Ctrl Pts',(-6.09007800846524,5.14985321596029,8.30647583195487));
#28834=CARTESIAN_POINT('Ctrl Pts',(-6.07032848755029,3.68356570204834,9.05261689300285));
#28835=CARTESIAN_POINT('Ctrl Pts',(-6.05057896663535,2.12808598853988,9.40459326154099));
#28836=CARTESIAN_POINT('Ctrl Pts',(-6.0308294457204,0.572606275031421,9.75656963007913));
#28837=CARTESIAN_POINT('Ctrl Pts',(-6.01107992480545,-1.07206563807355,
9.71438130610743));
#28838=CARTESIAN_POINT('Ctrl Pts',(-5.99133040389051,-2.60745410663262,
9.28311949031393));
#28839=CARTESIAN_POINT('Ctrl Pts',(-5.97158088297557,-4.1428425751917,8.85185767452044));
#28840=CARTESIAN_POINT('Ctrl Pts',(-5.95183136206062,-5.5689475992049,8.03152236690513));
#28841=CARTESIAN_POINT('Ctrl Pts',(-5.93208184114568,-6.71366973987204,
6.92110995531557));
#28842=CARTESIAN_POINT('Ctrl Pts',(-5.91233232023073,-7.85839188053918,
5.810697543726));
#28843=CARTESIAN_POINT('Ctrl Pts',(-5.89258279931578,-8.72173113786027,
4.41020802816217));
#28844=CARTESIAN_POINT('Ctrl Pts',(-5.87283327840084,-9.19950149525361,
2.88864962023233));
#28845=CARTESIAN_POINT('Ctrl Pts',(-5.86072749821325,-9.49235836766379,
1.9559864073723));
#28846=CARTESIAN_POINT('Ctrl Pts',(-5.84862171802566,-9.64034658300698,
0.977834339335062));
#28847=CARTESIAN_POINT('Ctrl Pts',(-5.83651593783807,-9.6409035792506,-0.000152919944957977));
#28848=CARTESIAN_POINT('Origin',(-3.5,0.,0.));
#28849=CARTESIAN_POINT('',(-5.08651593783807,-9.64135114576405,0.000239874805416028));
#28850=CARTESIAN_POINT('',(-5.28848406216194,-9.64152836430215,-0.000244200588832011));
#28851=CARTESIAN_POINT('',(-3.5,-9.64155,-1.18074933463192E-15));
#28852=CARTESIAN_POINT('Ctrl Pts',(-5.28848406216194,-9.64152836430215,
-0.000244200588832011));
#28853=CARTESIAN_POINT('Ctrl Pts',(-5.30359426693543,-9.64029754505796,
1.2202338220874));
#28854=CARTESIAN_POINT('Ctrl Pts',(-5.31870447170893,-9.40769088764861,
2.44116766783866));
#28855=CARTESIAN_POINT('Ctrl Pts',(-5.33381467648243,-8.95537463172337,
3.57440762075094));
#28856=CARTESIAN_POINT('Ctrl Pts',(-5.35356419739738,-8.36418281860958,
5.0555884840934));
#28857=CARTESIAN_POINT('Ctrl Pts',(-5.37331371831232,-7.39765393457124,
6.38695901098043));
#28858=CARTESIAN_POINT('Ctrl Pts',(-5.39306323922727,-6.17242670938371,
7.40785212805192));
#28859=CARTESIAN_POINT('Ctrl Pts',(-5.41281276014221,-4.94719948419616,
8.42874524512343));
#28860=CARTESIAN_POINT('Ctrl Pts',(-5.43256228105716,-3.46327391785939,
9.1391609523794));
#28861=CARTESIAN_POINT('Ctrl Pts',(-5.4523118019721,-1.89972711401413,9.45336773462645));
#28862=CARTESIAN_POINT('Ctrl Pts',(-5.47206132288705,-0.336180310168875,
9.76757451687349));
#28863=CARTESIAN_POINT('Ctrl Pts',(-5.49181084380199,1.30698773118489,9.6855723741116));
#28864=CARTESIAN_POINT('Ctrl Pts',(-5.51156036471694,2.83148285007319,9.2172571572859));
#28865=CARTESIAN_POINT('Ctrl Pts',(-5.53130988563188,4.35597796896149,8.74894194046021));
#28866=CARTESIAN_POINT('Ctrl Pts',(-5.55105940654683,5.76180016538431,7.89431364957073));
#28867=CARTESIAN_POINT('Ctrl Pts',(-5.57080892746177,6.8792976907094,6.7565070795787));
#28868=CARTESIAN_POINT('Ctrl Pts',(-5.59055844837672,7.99679521603447,5.61870050958668));
#28869=CARTESIAN_POINT('Ctrl Pts',(-5.61030796929166,8.8259680702618,4.1977156604921));
#28870=CARTESIAN_POINT('Ctrl Pts',(-5.6300574902066,9.26675336848597,2.66503407885353));
#28871=CARTESIAN_POINT('Ctrl Pts',(-5.64980701112155,9.70753866671014,1.13235249721493));
#28872=CARTESIAN_POINT('Ctrl Pts',(-5.6695565320365,9.75993640893116,-0.512025816967684));
#28873=CARTESIAN_POINT('Ctrl Pts',(-5.68930605295145,9.41762334273858,-2.06966065046962));
#28874=CARTESIAN_POINT('Ctrl Pts',(-5.70905557386639,9.07531027654599,-3.62729548397154));
#28875=CARTESIAN_POINT('Ctrl Pts',(-5.72880509478133,8.33828640193982,-5.09818683679275));
#28876=CARTESIAN_POINT('Ctrl Pts',(-5.74855461569628,7.29549425335211,-6.30483054753282));
#28877=CARTESIAN_POINT('Ctrl Pts',(-5.76830413661122,6.2527021047644,-7.51147425827288));
#28878=CARTESIAN_POINT('Ctrl Pts',(-5.78805365752617,4.90414168219518,-8.45387032693178));
#28879=CARTESIAN_POINT('Ctrl Pts',(-5.80780317844112,3.41255450047279,-9.01829232255752));
#28880=CARTESIAN_POINT('Ctrl Pts',(-5.82755269935606,1.92096731875038,-9.58271431818327));
#28881=CARTESIAN_POINT('Ctrl Pts',(-5.847302220271,0.286353377874808,-9.76916224077585));
#28882=CARTESIAN_POINT('Ctrl Pts',(-5.86705174118594,-1.29402545353786,
-9.5551359362069));
#28883=CARTESIAN_POINT('Ctrl Pts',(-5.88680126210089,-2.87440428495053,
-9.34110963163796));
#28884=CARTESIAN_POINT('Ctrl Pts',(-5.90655078301584,-4.4005480069003,-8.72660909990748));
#28885=CARTESIAN_POINT('Ctrl Pts',(-5.92630030393079,-5.68828471503698,
-7.78579100891321));
#28886=CARTESIAN_POINT('Ctrl Pts',(-5.94604982484573,-6.97602142317366,
-6.84497291791894));
#28887=CARTESIAN_POINT('Ctrl Pts',(-5.96579934576067,-8.02535111749725,
-5.57783726766087));
#28888=CARTESIAN_POINT('Ctrl Pts',(-5.98554886667561,-8.70964283572328,
-4.1372993979081));
#28889=CARTESIAN_POINT('Ctrl Pts',(-6.00319393183772,-9.32101827161303,
-2.85026136342924));
#28890=CARTESIAN_POINT('Ctrl Pts',(-6.02083899699983,-9.64100584945367,
-1.42480676785808));
#28891=CARTESIAN_POINT('Ctrl Pts',(-6.03848406216193,-9.6421289025524,0.00016016297285322));
#28892=CARTESIAN_POINT('Ctrl Pts',(-5.83651593783807,-9.6409035792506,-0.000152919944957977));
#28893=CARTESIAN_POINT('Ctrl Pts',(-5.82887219711071,-9.64125527363182,
-0.6176662837061));
#28894=CARTESIAN_POINT('Ctrl Pts',(-5.82122845638336,-9.58282883544997,
-1.23511394122783));
#28895=CARTESIAN_POINT('Ctrl Pts',(-5.81358471565601,-9.46497918425804,
-1.84100337620655));
#28896=CARTESIAN_POINT('Ctrl Pts',(-5.79383519474106,-9.16048505840356,
-3.4064706644198));
#28897=CARTESIAN_POINT('Ctrl Pts',(-5.77408567382611,-8.459295349229,-4.89477794055051));
#28898=CARTESIAN_POINT('Ctrl Pts',(-5.75433615291117,-7.44602819734076,
-6.12631932517789));
#28899=CARTESIAN_POINT('Ctrl Pts',(-5.73458663199622,-6.43276104545249,
-7.35786070980529));
#28900=CARTESIAN_POINT('Ctrl Pts',(-5.71483711108128,-5.10741645085051,
-8.33263620292937));
#28901=CARTESIAN_POINT('Ctrl Pts',(-5.69508759016634,-3.62993428970603,
-8.93301189084948));
#28902=CARTESIAN_POINT('Ctrl Pts',(-5.67533806925139,-2.15245212856156,
-9.53338757876959));
#28903=CARTESIAN_POINT('Ctrl Pts',(-5.65558854833645,-0.522832400874613,
-9.75936346148576));
#28904=CARTESIAN_POINT('Ctrl Pts',(-5.6358390274215,1.06226571617635,-9.58366923145192));
#28905=CARTESIAN_POINT('Ctrl Pts',(-5.61608950650656,2.6473638332273,-9.40797500141808));
#28906=CARTESIAN_POINT('Ctrl Pts',(-5.59633998559161,4.18794033964224,-8.83061065863424));
#28907=CARTESIAN_POINT('Ctrl Pts',(-5.57659046467667,5.49808161214777,-7.92125135163658));
#28908=CARTESIAN_POINT('Ctrl Pts',(-5.55684094376172,6.80822288465331,-7.01189204463891));
#28909=CARTESIAN_POINT('Ctrl Pts',(-5.53709142284678,7.88792892324943,-5.77053777342741));
#28910=CARTESIAN_POINT('Ctrl Pts',(-5.51734190193183,8.60690301052564,-4.3469926336545));
#28911=CARTESIAN_POINT('Ctrl Pts',(-5.49759238101689,9.32587709780184,-2.92344749388162));
#28912=CARTESIAN_POINT('Ctrl Pts',(-5.47784286010194,9.68411923375813,-1.31771148554732));
#28913=CARTESIAN_POINT('Ctrl Pts',(-5.458093339187,9.63839748980967,0.276438452593999));
#28914=CARTESIAN_POINT('Ctrl Pts',(-5.43834381827205,9.5926757458612,1.87058839073534));
#28915=CARTESIAN_POINT('Ctrl Pts',(-5.41859429735711,9.14299012200796,3.4531522586837));
#28916=CARTESIAN_POINT('Ctrl Pts',(-5.39884477644216,8.34360776000916,4.83314948421386));
#28917=CARTESIAN_POINT('Ctrl Pts',(-5.37909525552722,7.54422539801037,6.21314670974401));
#28918=CARTESIAN_POINT('Ctrl Pts',(-5.35934573461227,6.39514629786602,7.39057729285595));
#28919=CARTESIAN_POINT('Ctrl Pts',(-5.33959621369733,5.03503897622948,8.22335131789296));
#28920=CARTESIAN_POINT('Ctrl Pts',(-5.31984669278238,3.67493165459292,9.05612534292997));
#28921=CARTESIAN_POINT('Ctrl Pts',(-5.30009717186744,2.10379611146416,9.54424280989203));
#28922=CARTESIAN_POINT('Ctrl Pts',(-5.28034765095249,0.511233772193015,
9.62879870076278));
#28923=CARTESIAN_POINT('Ctrl Pts',(-5.26059813003755,-1.08132856707812,
9.71335459163353));
#28924=CARTESIAN_POINT('Ctrl Pts',(-5.24084860912261,-2.69531770249161,
9.39434890641299));
#28925=CARTESIAN_POINT('Ctrl Pts',(-5.22109908820766,-4.13596072478972,
8.71027859902533));
#28926=CARTESIAN_POINT('Ctrl Pts',(-5.20134956729271,-5.57660374708781,
8.02620829163769));
#28927=CARTESIAN_POINT('Ctrl Pts',(-5.18160004637777,-6.8439006562705,6.97707336208295));
#28928=CARTESIAN_POINT('Ctrl Pts',(-5.16185052546282,-7.78491665217157,
5.68948126883141));
#28929=CARTESIAN_POINT('Ctrl Pts',(-5.14210100454788,-8.72593264807268,
4.40188917557982));
#28930=CARTESIAN_POINT('Ctrl Pts',(-5.12235148363294,-9.34066773069216,
2.87583991863138));
#28931=CARTESIAN_POINT('Ctrl Pts',(-5.10260196271799,-9.55493692701037,
1.2954940024931));
#28932=CARTESIAN_POINT('Ctrl Pts',(-5.09723995442469,-9.61311115881104,
0.866429016809633));
#28933=CARTESIAN_POINT('Ctrl Pts',(-5.09187794613138,-9.64176600192921,
0.433361682257971));
#28934=CARTESIAN_POINT('Ctrl Pts',(-5.08651593783807,-9.64135114576405,
0.000239874805416028));
#28935=CARTESIAN_POINT('Origin',(-3.5,0.,0.));
#28936=CARTESIAN_POINT('',(-4.33651593783807,-9.64225279696581,-0.000111202327370922));
#28937=CARTESIAN_POINT('',(-4.53848406216194,-9.64081637547245,0.000107710467356636));
#28938=CARTESIAN_POINT('',(-3.5,-9.64155,-1.18074933463192E-15));
#28939=CARTESIAN_POINT('Ctrl Pts',(-4.53848406216194,-9.64081637547245,
0.000107710467356636));
#28940=CARTESIAN_POINT('Ctrl Pts',(-4.54685049504115,-9.64108436120108,
0.676022573073167));
#28941=CARTESIAN_POINT('Ctrl Pts',(-4.55521692792037,-9.57099666503678,
1.35188265298491));
#28942=CARTESIAN_POINT('Ctrl Pts',(-4.56358336079958,-9.42998123846142,
2.01260489815126));
#28943=CARTESIAN_POINT('Ctrl Pts',(-4.58333288171452,-9.09710495095793,
3.57228367502892));
#28944=CARTESIAN_POINT('Ctrl Pts',(-4.60308240262947,-8.36899991173037,
5.04761028815404));
#28945=CARTESIAN_POINT('Ctrl Pts',(-4.62283192354442,-7.33353234839077,
6.26054533797998));
#28946=CARTESIAN_POINT('Ctrl Pts',(-4.64258144445936,-6.29806478505116,
7.47348038780594));
#28947=CARTESIAN_POINT('Ctrl Pts',(-4.6623309653743,-4.95523469759951,8.42402387433271));
#28948=CARTESIAN_POINT('Ctrl Pts',(-4.68208048628925,-3.46709207573716,
8.99746615287645));
#28949=CARTESIAN_POINT('Ctrl Pts',(-4.70183000720419,-1.97894945387482,
9.57090843142019));
#28950=CARTESIAN_POINT('Ctrl Pts',(-4.72157952811914,-0.345494297601781,
9.7672495019809));
#28951=CARTESIAN_POINT('Ctrl Pts',(-4.74132904903409,1.23615136422273,9.56279532555869));
#28952=CARTESIAN_POINT('Ctrl Pts',(-4.76107856994903,2.81779702604719,9.35834114913648));
#28953=CARTESIAN_POINT('Ctrl Pts',(-4.78082809086397,4.34763319342313,8.75309172573136));
#28954=CARTESIAN_POINT('Ctrl Pts',(-4.80057761177892,5.64104236523506,7.82008731840125));
#28955=CARTESIAN_POINT('Ctrl Pts',(-4.82032713269386,6.93445153704702,6.88708291107111));
#28956=CARTESIAN_POINT('Ctrl Pts',(-4.84007665360881,7.99143371329496,5.62632351981596));
#28957=CARTESIAN_POINT('Ctrl Pts',(-4.85982617452376,8.6844344458204,4.18995501050368));
#28958=CARTESIAN_POINT('Ctrl Pts',(-4.8795756954387,9.37743517834584,2.75358650119141));
#28959=CARTESIAN_POINT('Ctrl Pts',(-4.89932521635364,9.70645446714877,1.141608873822));
#28960=CARTESIAN_POINT('Ctrl Pts',(-4.91907473726859,9.63178693709627,-0.451447707025219));
#28961=CARTESIAN_POINT('Ctrl Pts',(-4.93882425818353,9.55711940704377,-2.04450428787242));
#28962=CARTESIAN_POINT('Ctrl Pts',(-4.95857377909848,9.07876505813585,-3.61863982219743));
#28963=CARTESIAN_POINT('Ctrl Pts',(-4.97832330001343,8.25445071526159,-4.98389085184599));
#28964=CARTESIAN_POINT('Ctrl Pts',(-4.99807282092837,7.43013637238733,-6.34914188149456));
#28965=CARTESIAN_POINT('Ctrl Pts',(-5.01782234184331,6.25986203554674,-7.50550840646669));
#28966=CARTESIAN_POINT('Ctrl Pts',(-5.03757186275826,4.8848540192266,-8.31344247857905));
#28967=CARTESIAN_POINT('Ctrl Pts',(-5.0573213836732,3.50984600290644,-9.12137655069141));
#28968=CARTESIAN_POINT('Ctrl Pts',(-5.07707090458815,1.93010430710673,-9.580878169944));
#28969=CARTESIAN_POINT('Ctrl Pts',(-5.0968204255031,0.336268930087386,-9.63649562032042));
#28970=CARTESIAN_POINT('Ctrl Pts',(-5.11656994641804,-1.25756644693194,
-9.69211307069684));
#28971=CARTESIAN_POINT('Ctrl Pts',(-5.13631946733298,-2.86549550517089,
-9.34384635219709));
#28972=CARTESIAN_POINT('Ctrl Pts',(-5.15606898824793,-4.29347665309604,
-8.63372358042091));
#28973=CARTESIAN_POINT('Ctrl Pts',(-5.17581850916287,-5.72145780102118,
-7.92360080864472));
#28974=CARTESIAN_POINT('Ctrl Pts',(-5.19556803007782,-6.96949103863252,
-6.8516219835921));
#28975=CARTESIAN_POINT('Ctrl Pts',(-5.21531755099276,-7.88696626626681,
-5.54715131834045));
#28976=CARTESIAN_POINT('Ctrl Pts',(-5.23506707190771,-8.80444149390112,
-4.24268065308877));
#28977=CARTESIAN_POINT('Ctrl Pts',(-5.25481659282265,-9.39135871155838,
-2.70571814763806));
#28978=CARTESIAN_POINT('Ctrl Pts',(-5.2745661137376,-9.57688994929239,-1.12174129501374));
#28979=CARTESIAN_POINT('Ctrl Pts',(-5.27920542987904,-9.62047268072516,
-0.749652806806595));
#28980=CARTESIAN_POINT('Ctrl Pts',(-5.28384474602049,-9.64190626517592,
-0.374969988608132));
#28981=CARTESIAN_POINT('Ctrl Pts',(-5.28848406216194,-9.64152836430215,
-0.000244200588832011));
#28982=CARTESIAN_POINT('Ctrl Pts',(-5.08651593783807,-9.64135114576405,
0.000239874805416028));
#28983=CARTESIAN_POINT('Ctrl Pts',(-5.07212842521643,-9.64023799039654,
-1.16192644992957));
#28984=CARTESIAN_POINT('Ctrl Pts',(-5.05774091259479,-9.42983072252804,
-2.32448496508033));
#28985=CARTESIAN_POINT('Ctrl Pts',(-5.04335339997315,-9.01881669295193,
-3.41116839932792));
#28986=CARTESIAN_POINT('Ctrl Pts',(-5.02360387905821,-8.45462395255836,
-4.90284230968261));
#28987=CARTESIAN_POINT('Ctrl Pts',(-5.00385435814326,-7.51243516175428,
-6.2515475550639));
#28988=CARTESIAN_POINT('Ctrl Pts',(-4.98410483722832,-6.30595173762386,
-7.29452514372254));
#28989=CARTESIAN_POINT('Ctrl Pts',(-4.96435531631337,-5.09946831349343,
-8.3375027323812));
#28990=CARTESIAN_POINT('Ctrl Pts',(-4.94460579539843,-3.62869025603665,
-9.0747526643172));
#28991=CARTESIAN_POINT('Ctrl Pts',(-4.92485627448348,-2.07110805440109,
-9.41730512496206));
#28992=CARTESIAN_POINT('Ctrl Pts',(-4.90510675356854,-0.513525852765532,
-9.75985758560692));
#28993=CARTESIAN_POINT('Ctrl Pts',(-4.88535723265359,1.13086049304882,-9.70771257496064));
#28994=CARTESIAN_POINT('Ctrl Pts',(-4.86560771173865,2.66360980057637,-9.26716284630389));
#28995=CARTESIAN_POINT('Ctrl Pts',(-4.8458581908237,4.19635910810388,-8.82661311764716));
#28996=CARTESIAN_POINT('Ctrl Pts',(-4.82610866990876,5.61747137734461,-7.99765867097999));
#28997=CARTESIAN_POINT('Ctrl Pts',(-4.80635914899381,6.75544968493727,-6.88033603422992));
#28998=CARTESIAN_POINT('Ctrl Pts',(-4.78660962807887,7.89342799252996,-5.76301339747983));
#28999=CARTESIAN_POINT('Ctrl Pts',(-4.76686010716393,8.74827233847458,-4.35732257064681));
#29000=CARTESIAN_POINT('Ctrl Pts',(-4.74711058624898,9.2168218547275,-2.83289944894966));
#29001=CARTESIAN_POINT('Ctrl Pts',(-4.72736106533404,9.68537137098043,-1.3084763272525));
#29002=CARTESIAN_POINT('Ctrl Pts',(-4.70761154441909,9.76762605754167,0.334679089308759));
#29003=CARTESIAN_POINT('Ctrl Pts',(-4.68786202350414,9.45365958699668,1.89827416429438));
#29004=CARTESIAN_POINT('Ctrl Pts',(-4.6681125025892,9.1396931164517,3.46186923927994));
#29005=CARTESIAN_POINT('Ctrl Pts',(-4.64836298167426,8.42950548880053,4.94590397268984));
#29006=CARTESIAN_POINT('Ctrl Pts',(-4.62861346075931,7.40880069505612,6.17128808682416));
#29007=CARTESIAN_POINT('Ctrl Pts',(-4.60886393984437,6.38809590131167,7.39667220095852));
#29008=CARTESIAN_POINT('Ctrl Pts',(-4.58911441892942,5.05687394147397,8.36340569581729));
#29009=CARTESIAN_POINT('Ctrl Pts',(-4.56936489801448,3.57578396013533,8.95482514960961));
#29010=CARTESIAN_POINT('Ctrl Pts',(-4.54961537709953,2.09469397879668,9.54624460340193));
#29011=CARTESIAN_POINT('Ctrl Pts',(-4.52986585618459,0.463735975957077,
9.76235001612781));
#29012=CARTESIAN_POINT('Ctrl Pts',(-4.51011633526964,-1.12026937089548,
9.57706222838065));
#29013=CARTESIAN_POINT('Ctrl Pts',(-4.4903668143547,-2.70427471774801,9.39177444063348));
#29014=CARTESIAN_POINT('Ctrl Pts',(-4.47061729343975,-4.24132740861351,
8.80509345241328));
#29015=CARTESIAN_POINT('Ctrl Pts',(-4.45086777252481,-5.54593906707505,
7.88781872598075));
#29016=CARTESIAN_POINT('Ctrl Pts',(-4.43111825160986,-6.85055072553659,
6.97054399954821));
#29017=CARTESIAN_POINT('Ctrl Pts',(-4.41136873069492,-7.92272135159418,
5.72267553490333));
#29018=CARTESIAN_POINT('Ctrl Pts',(-4.39161920977997,-8.63306358601724,
4.2948035472446));
#29019=CARTESIAN_POINT('Ctrl Pts',(-4.373251452466,-9.29370714430582,2.96683178237609));
#29020=CARTESIAN_POINT('Ctrl Pts',(-4.35488369515204,-9.64138137487533,
1.48316305483911));
#29021=CARTESIAN_POINT('Ctrl Pts',(-4.33651593783807,-9.64225279696581,
-0.000111202327370922));
#29022=CARTESIAN_POINT('Origin',(-3.5,0.,0.));
#29023=CARTESIAN_POINT('',(-3.58651593783807,-9.64084195522704,-0.000123447406648672));
#29024=CARTESIAN_POINT('',(-3.78848406216194,-9.64221558294609,0.000128484054292971));
#29025=CARTESIAN_POINT('',(-3.5,-9.64155,-1.18074933463192E-15));
#29026=CARTESIAN_POINT('Ctrl Pts',(-3.78848406216194,-9.64221558294609,
0.000128484054292971));
#29027=CARTESIAN_POINT('Ctrl Pts',(-3.79010672314687,-9.64230233742042,
0.131166705674271));
#29028=CARTESIAN_POINT('Ctrl Pts',(-3.7917293841318,-9.63968591491053,0.262201459667352));
#29029=CARTESIAN_POINT('Ctrl Pts',(-3.79335204511673,-9.63434364026827,
0.393124986510688));
#29030=CARTESIAN_POINT('Ctrl Pts',(-3.81310156603167,-9.56932244005419,
1.98660443518506));
#29031=CARTESIAN_POINT('Ctrl Pts',(-3.83285108694662,-9.10050726460994,
3.56360725535284));
#29032=CARTESIAN_POINT('Ctrl Pts',(-3.85260060786156,-8.28447377087269,
4.93382397066609));
#29033=CARTESIAN_POINT('Ctrl Pts',(-3.87235012877651,-7.46844027713545,
6.30404068597931));
#29034=CARTESIAN_POINT('Ctrl Pts',(-3.89209964969145,-6.30518846510522,
7.46747129643801));
#29035=CARTESIAN_POINT('Ctrl Pts',(-3.9118491706064,-4.93509718533139,8.28371537446398));
#29036=CARTESIAN_POINT('Ctrl Pts',(-3.93159869152134,-3.56500590555757,
9.09995945248994));
#29037=CARTESIAN_POINT('Ctrl Pts',(-3.95134821243629,-1.98807515804016,
9.56901699808319));
#29038=CARTESIAN_POINT('Ctrl Pts',(-3.97109773335123,-0.394605721546979,
9.63428310557247));
#29039=CARTESIAN_POINT('Ctrl Pts',(-3.99084725426618,1.1988637149462,9.69954921306175));
#29040=CARTESIAN_POINT('Ctrl Pts',(-4.01059677518112,2.80887184041515,9.36102388244707));
#29041=CARTESIAN_POINT('Ctrl Pts',(-4.03034629609607,4.24112616574349,8.65955965855324));
#29042=CARTESIAN_POINT('Ctrl Pts',(-4.05009581701101,5.67338049107185,7.95809543465941));
#29043=CARTESIAN_POINT('Ctrl Pts',(-4.06984533792595,6.92788101625959,6.89369231748643));
#29044=CARTESIAN_POINT('Ctrl Pts',(-4.0895948588409,7.85323718260037,5.59480029917241));
#29045=CARTESIAN_POINT('Ctrl Pts',(-4.10934437975584,8.77859334894114,4.29590828085841));
#29046=CARTESIAN_POINT('Ctrl Pts',(-4.12909390067079,9.37480515643494,2.76252736140337));
#29047=CARTESIAN_POINT('Ctrl Pts',(-4.14884342158574,9.56992298303575,1.17970281535688));
#29048=CARTESIAN_POINT('Ctrl Pts',(-4.16859294250068,9.76504080963655,-0.403121730689601));
#29049=CARTESIAN_POINT('Ctrl Pts',(-4.18834246341562,9.55906465534435,-2.03538990332756));
#29050=CARTESIAN_POINT('Ctrl Pts',(-4.20809198433057,8.97685130136602,-3.52012291645618));
#29051=CARTESIAN_POINT('Ctrl Pts',(-4.22784150524551,8.39463794738768,-5.00485592958482));
#29052=CARTESIAN_POINT('Ctrl Pts',(-4.24759102616046,7.43618739372319,-6.34205378320413));
#29053=CARTESIAN_POINT('Ctrl Pts',(-4.26734054707541,6.21716349375353,-7.37034617407725));
#29054=CARTESIAN_POINT('Ctrl Pts',(-4.28709006799035,4.99813959378387,-8.39863856495036));
#29055=CARTESIAN_POINT('Ctrl Pts',(-4.30683958890529,3.51854234750906,-9.11802549307728));
#29056=CARTESIAN_POINT('Ctrl Pts',(-4.32658910982024,1.95692652575344,-9.44169281467044));
#29057=CARTESIAN_POINT('Ctrl Pts',(-4.34633863073518,0.395310703997839,
-9.7653601362636));
#29058=CARTESIAN_POINT('Ctrl Pts',(-4.36608815165013,-1.24832369323855,
-9.69330785132303));
#29059=CARTESIAN_POINT('Ctrl Pts',(-4.38583767256508,-2.7756262271073,-9.23423108229325));
#29060=CARTESIAN_POINT('Ctrl Pts',(-4.40558719348002,-4.30292876097604,
-8.77515431326348));
#29061=CARTESIAN_POINT('Ctrl Pts',(-4.42533671439496,-5.71389943147713,
-7.9290530601445));
#29062=CARTESIAN_POINT('Ctrl Pts',(-4.44508623530991,-6.83826518265192,
-6.7980330924119));
#29063=CARTESIAN_POINT('Ctrl Pts',(-4.46483575622485,-7.96263093382673,
-5.66701312467929));
#29064=CARTESIAN_POINT('Ctrl Pts',(-4.4845852771398,-8.80039176567523,-4.25107444233305));
#29065=CARTESIAN_POINT('Ctrl Pts',(-4.50433479805475,-9.25044841370977,
-2.72108963084481));
#29066=CARTESIAN_POINT('Ctrl Pts',(-4.51571788609048,-9.50984885525497,
-1.83924789516393));
#29067=CARTESIAN_POINT('Ctrl Pts',(-4.52710097412621,-9.64045176307607,
-0.919519387099601));
#29068=CARTESIAN_POINT('Ctrl Pts',(-4.53848406216194,-9.64081637547245,
0.000107710467356636));
#29069=CARTESIAN_POINT('Ctrl Pts',(-4.33651593783807,-9.64225279696581,
-0.000111202327370922));
#29070=CARTESIAN_POINT('Ctrl Pts',(-4.33513417423709,-9.64231835201998,
-0.111694469886249));
#29071=CARTESIAN_POINT('Ctrl Pts',(-4.33375241063611,-9.64042127976813,
-0.223275505057436));
#29072=CARTESIAN_POINT('Ctrl Pts',(-4.33237064703514,-9.63654717632921,
-0.334787855250616));
#29073=CARTESIAN_POINT('Ctrl Pts',(-4.31262112612019,-9.58117468942955,
-1.92863175941445));
#29074=CARTESIAN_POINT('Ctrl Pts',(-4.29287160520524,-9.12191587284169,
-3.50844405706951));
#29075=CARTESIAN_POINT('Ctrl Pts',(-4.2731220842903,-8.31419314165281,-4.88357622986835));
#29076=CARTESIAN_POINT('Ctrl Pts',(-4.25337256337535,-7.50647041046394,
-6.25870840266719));
#29077=CARTESIAN_POINT('Ctrl Pts',(-4.23362304246041,-6.35028376467405,
-7.42916045060979));
#29078=CARTESIAN_POINT('Ctrl Pts',(-4.21387352154547,-4.98515944501452,
-8.25368461339688));
#29079=CARTESIAN_POINT('Ctrl Pts',(-4.19412400063052,-3.62003512535496,
-9.07820877618398));
#29080=CARTESIAN_POINT('Ctrl Pts',(-4.17437447971558,-2.04597313182576,
-9.55680505381556));
#29081=CARTESIAN_POINT('Ctrl Pts',(-4.15462495880063,-0.452928047828257,
-9.63171742593875));
#29082=CARTESIAN_POINT('Ctrl Pts',(-4.13487543788569,1.14011703616925,-9.70662979806195));
#29083=CARTESIAN_POINT('Ctrl Pts',(-4.11512591697074,2.75214521063503,-9.37785826467676));
#29084=CARTESIAN_POINT('Ctrl Pts',(-4.0953763960558,4.18862021106955,-8.6850783022988));
#29085=CARTESIAN_POINT('Ctrl Pts',(-4.07562687514085,5.62509521150404,-7.99229833992086));
#29086=CARTESIAN_POINT('Ctrl Pts',(-4.05587735422591,6.88601703790726,-6.93550994855018));
#29087=CARTESIAN_POINT('Ctrl Pts',(-4.03612783331096,7.81922022206973,-5.64224419078239));
#29088=CARTESIAN_POINT('Ctrl Pts',(-4.01637831239602,8.75242340623219,-4.34897843301462));
#29089=CARTESIAN_POINT('Ctrl Pts',(-3.99662879148107,9.35790794815393,-2.8192353088497));
#29090=CARTESIAN_POINT('Ctrl Pts',(-3.97687927056613,9.56260521115508,-1.23762109113875));
#29091=CARTESIAN_POINT('Ctrl Pts',(-3.95712974965118,9.76730247415624,0.343993126572243));
#29092=CARTESIAN_POINT('Ctrl Pts',(-3.93738022873624,9.57121245823682,1.97747843782926));
#29093=CARTESIAN_POINT('Ctrl Pts',(-3.91763070782129,8.99799890563587,3.46570917473141));
#29094=CARTESIAN_POINT('Ctrl Pts',(-3.89788118690635,8.42478535303492,4.95393991163352));
#29095=CARTESIAN_POINT('Ctrl Pts',(-3.8781316659914,7.47444826375242,6.29691607418075));
#29096=CARTESIAN_POINT('Ctrl Pts',(-3.85838214507646,6.26167237487477,7.33257004462774));
#29097=CARTESIAN_POINT('Ctrl Pts',(-3.83863262416151,5.04889648599708,8.36822401507476));
#29098=CARTESIAN_POINT('Ctrl Pts',(-3.81888310324657,3.57368179752421,9.09655579342157));
#29099=CARTESIAN_POINT('Ctrl Pts',(-3.79913358233162,2.01405420216457,9.42967178964279));
#29100=CARTESIAN_POINT('Ctrl Pts',(-3.77938406141668,0.454426606804935,
9.762787785864));
#29101=CARTESIAN_POINT('Ctrl Pts',(-3.75963454050173,-1.18961389544146,
9.7006879999596));
#29102=CARTESIAN_POINT('Ctrl Pts',(-3.73988501958679,-2.71966785780379,
9.25086650713709));
#29103=CARTESIAN_POINT('Ctrl Pts',(-3.72013549867184,-4.2497218201661,8.80104501431459));
#29104=CARTESIAN_POINT('Ctrl Pts',(-3.7003859777569,-5.66578924264433,7.96350181457399));
#29105=CARTESIAN_POINT('Ctrl Pts',(-3.68063645684195,-6.79698200367094,
6.83930990900508));
#29106=CARTESIAN_POINT('Ctrl Pts',(-3.66088693592701,-7.92817476469756,
5.71511800343617));
#29107=CARTESIAN_POINT('Ctrl Pts',(-3.64113741501206,-8.77449286427254,
4.30427739203897));
#29108=CARTESIAN_POINT('Ctrl Pts',(-3.62138789409712,-9.23380436433331,
2.77704543550532));
#29109=CARTESIAN_POINT('Ctrl Pts',(-3.60976390867744,-9.50414156404529,
1.87816175768467));
#29110=CARTESIAN_POINT('Ctrl Pts',(-3.59813992325775,-9.64041378177036,
0.938958344725818));
#29111=CARTESIAN_POINT('Ctrl Pts',(-3.58651593783807,-9.64084195522704,
-0.000123447406648672));
#29112=CARTESIAN_POINT('Origin',(-3.5,0.,0.));
#29113=CARTESIAN_POINT('',(-2.83651593783807,-9.64146833476739,0.000244149912687573));
#29114=CARTESIAN_POINT('',(-3.03848406216193,-9.6414091844932,-0.000242700028759701));
#29115=CARTESIAN_POINT('',(-3.5,-9.64155,-1.18074933463192E-15));
#29116=CARTESIAN_POINT('Ctrl Pts',(-3.03848406216193,-9.6414091844932,-0.000242700028759701));
#29117=CARTESIAN_POINT('Ctrl Pts',(-3.05311247216753,-9.64025195196911,
1.18136192116153));
#29118=CARTESIAN_POINT('Ctrl Pts',(-3.06774088217312,-9.42257645101838,
2.36338120258475));
#29119=CARTESIAN_POINT('Ctrl Pts',(-3.08236929217871,-8.99799891745031,
3.46570917928206));
#29120=CARTESIAN_POINT('Ctrl Pts',(-3.10211881309366,-8.42478536409669,
4.95393991813827));
#29121=CARTESIAN_POINT('Ctrl Pts',(-3.1218683340086,-7.47444827356636,6.2969160824488));
#29122=CARTESIAN_POINT('Ctrl Pts',(-3.14161785492354,-6.26167238309626,
7.33257005425562));
#29123=CARTESIAN_POINT('Ctrl Pts',(-3.16136737583849,-5.0488964926262,8.36822402606241));
#29124=CARTESIAN_POINT('Ctrl Pts',(-3.18111689675343,-3.57368180221639,
9.0965558053655));
#29125=CARTESIAN_POINT('Ctrl Pts',(-3.20086641766838,-2.01405420480899,
9.42967180202408));
#29126=CARTESIAN_POINT('Ctrl Pts',(-3.22061593858332,-0.45442660740154,
9.76278779868267));
#29127=CARTESIAN_POINT('Ctrl Pts',(-3.24036545949827,1.1896138970035,9.70068801269671));
#29128=CARTESIAN_POINT('Ctrl Pts',(-3.26011498041321,2.71966786137481,9.25086651928357));
#29129=CARTESIAN_POINT('Ctrl Pts',(-3.27986450132816,4.24972182574611,8.80104502587043));
#29130=CARTESIAN_POINT('Ctrl Pts',(-3.2996140222431,5.66578925008368,7.9635018250301));
#29131=CARTESIAN_POINT('Ctrl Pts',(-3.31936354315805,6.79698201259557,6.83930991798508));
#29132=CARTESIAN_POINT('Ctrl Pts',(-3.33911306407299,7.92817477510741,5.7151180109401));
#29133=CARTESIAN_POINT('Ctrl Pts',(-3.35886258498794,8.77449287579359,4.30427739769045));
#29134=CARTESIAN_POINT('Ctrl Pts',(-3.37861210590288,9.23380437645742,2.77704543915155));
#29135=CARTESIAN_POINT('Ctrl Pts',(-3.39836162681783,9.69311587712127,1.24981348061261));
#29136=CARTESIAN_POINT('Ctrl Pts',(-3.41811114773277,9.76542077776275,-0.393809823215587));
#29137=CARTESIAN_POINT('Ctrl Pts',(-3.43786066864772,9.44199347079099,-1.9554753722144));
#29138=CARTESIAN_POINT('Ctrl Pts',(-3.45761018956266,9.11856616381923,-3.51714092121322));
#29139=CARTESIAN_POINT('Ctrl Pts',(-3.47735971047761,8.39940664923424,-4.99684871538265));
#29140=CARTESIAN_POINT('Ctrl Pts',(-3.49710923139255,7.37130162702222,-6.21603064320442));
#29141=CARTESIAN_POINT('Ctrl Pts',(-3.5168587523075,6.3431966048102,-7.43521257102619));
#29142=CARTESIAN_POINT('Ctrl Pts',(-3.53660827322244,5.00614607497117,-8.39386863250029));
#29143=CARTESIAN_POINT('Ctrl Pts',(-3.55635779413739,3.52150256200938,-8.97631017398341));
#29144=CARTESIAN_POINT('Ctrl Pts',(-3.57610731505233,2.03685904904759,-9.55875171546654));
#29145=CARTESIAN_POINT('Ctrl Pts',(-3.59585683596728,0.404622552963038,
-9.76497873695868));
#29146=CARTESIAN_POINT('Ctrl Pts',(-3.61560635688222,-1.1782319628052,-9.57010418311216));
#29147=CARTESIAN_POINT('Ctrl Pts',(-3.63535587779717,-2.76108647857339,
-9.37522962926565));
#29148=CARTESIAN_POINT('Ctrl Pts',(-3.65510539871212,-4.29455901402527,
-8.7792535000805));
#29149=CARTESIAN_POINT('Ctrl Pts',(-3.67485491962706,-5.59359323858005,
-7.85409697642628));
#29150=CARTESIAN_POINT('Ctrl Pts',(-3.694604440542,-6.89262746313484,-6.92894045277205));
#29151=CARTESIAN_POINT('Ctrl Pts',(-3.71435396145695,-7.95722337679252,
-5.67460353464874));
#29152=CARTESIAN_POINT('Ctrl Pts',(-3.73410348237189,-8.6589077211294,-4.24245703699665));
#29153=CARTESIAN_POINT('Ctrl Pts',(-3.7522303423019,-9.30294024625533,-2.92797862134267));
#29154=CARTESIAN_POINT('Ctrl Pts',(-3.77035720223192,-9.64124644261487,
-1.4637087011892));
#29155=CARTESIAN_POINT('Ctrl Pts',(-3.78848406216194,-9.64221558294609,
0.000128484054292971));
#29156=CARTESIAN_POINT('Ctrl Pts',(-3.58651593783807,-9.64084195522704,
-0.000123447406648672));
#29157=CARTESIAN_POINT('Ctrl Pts',(-3.57839040234281,-9.6411412620908,-0.656571486476391));
#29158=CARTESIAN_POINT('Ctrl Pts',(-3.57026486684754,-9.57506099308481,
-1.31296009608115));
#29159=CARTESIAN_POINT('Ctrl Pts',(-3.56213933135228,-9.44199345839355,
-1.95547536964678));
#29160=CARTESIAN_POINT('Ctrl Pts',(-3.54238981043734,-9.11856615184647,
-3.51714091659511));
#29161=CARTESIAN_POINT('Ctrl Pts',(-3.52264028952239,-8.39940663820575,
-4.99684870882167));
#29162=CARTESIAN_POINT('Ctrl Pts',(-3.50289076860745,-7.37130161734365,
-6.21603063504264));
#29163=CARTESIAN_POINT('Ctrl Pts',(-3.4831412476925,-6.34319659648157,-7.4352125612636));
#29164=CARTESIAN_POINT('Ctrl Pts',(-3.46339172677756,-5.00614606839814,
-8.39386862147897));
#29165=CARTESIAN_POINT('Ctrl Pts',(-3.44364220586261,-3.52150255738573,
-8.97631016219736));
#29166=CARTESIAN_POINT('Ctrl Pts',(-3.42389268494767,-2.03685904637332,
-9.55875170291574));
#29167=CARTESIAN_POINT('Ctrl Pts',(-3.40414316403272,-0.404622552431944,
-9.76497872413714));
#29168=CARTESIAN_POINT('Ctrl Pts',(-3.38439364311778,1.17823196125796,-9.57010417054653));
#29169=CARTESIAN_POINT('Ctrl Pts',(-3.36464412220284,2.76108647494785,-9.37522961695592));
#29170=CARTESIAN_POINT('Ctrl Pts',(-3.34489460128789,4.29455900838627,-8.77925348855332));
#29171=CARTESIAN_POINT('Ctrl Pts',(-3.32514508037294,5.59359323123543,-7.85409696611386));
#29172=CARTESIAN_POINT('Ctrl Pts',(-3.305395559458,6.89262745408462,-6.92894044367438));
#29173=CARTESIAN_POINT('Ctrl Pts',(-3.28564603854305,7.95722336634453,-5.67460352719801));
#29174=CARTESIAN_POINT('Ctrl Pts',(-3.26589651762811,8.65890770976012,-4.24245703142631));
#29175=CARTESIAN_POINT('Ctrl Pts',(-3.24614699671316,9.36059205317571,-2.81031053565461));
#29176=CARTESIAN_POINT('Ctrl Pts',(-3.22639747579822,9.69936482774697,-1.20035446058757));
#29177=CARTESIAN_POINT('Ctrl Pts',(-3.20664795488328,9.63434362761826,0.393124985994513));
#29178=CARTESIAN_POINT('Ctrl Pts',(-3.18689843396833,9.56932242748955,1.9866044325766));
#29179=CARTESIAN_POINT('Ctrl Pts',(-3.16714891305338,9.10050725266087,3.56360725067374));
#29180=CARTESIAN_POINT('Ctrl Pts',(-3.14739939213844,8.28447375999511,4.93382396418786));
#29181=CARTESIAN_POINT('Ctrl Pts',(-3.12764987122349,7.46844026732935,6.30404067770196));
#29182=CARTESIAN_POINT('Ctrl Pts',(-3.10790035030855,6.30518845682652,7.46747128663305));
#29183=CARTESIAN_POINT('Ctrl Pts',(-3.0881508293936,4.93509717885166,8.28371536358729));
#29184=CARTESIAN_POINT('Ctrl Pts',(-3.06840130847866,3.56500590087681,9.09995944054153));
#29185=CARTESIAN_POINT('Ctrl Pts',(-3.04865178756371,1.98807515542992,9.56901698551892));
#29186=CARTESIAN_POINT('Ctrl Pts',(-3.02890226664877,0.39460572102899,9.63428309292253));
#29187=CARTESIAN_POINT('Ctrl Pts',(-3.00915274573382,-1.19886371337197,
9.69954920032614));
#29188=CARTESIAN_POINT('Ctrl Pts',(-2.98940322481888,-2.80887183672698,
9.36102387015595));
#29189=CARTESIAN_POINT('Ctrl Pts',(-2.96965370390394,-4.24112616017478,
8.65955964718316));
#29190=CARTESIAN_POINT('Ctrl Pts',(-2.94990418298899,-5.67338048362257,
7.95809542421037));
#29191=CARTESIAN_POINT('Ctrl Pts',(-2.93015466207404,-6.92788100716316,
6.89369230843497));
#29192=CARTESIAN_POINT('Ctrl Pts',(-2.9104051411591,-7.85323717228894,5.59480029182642));
#29193=CARTESIAN_POINT('Ctrl Pts',(-2.89065562024415,-8.77859333741471,
4.29590827521789));
#29194=CARTESIAN_POINT('Ctrl Pts',(-2.87090609932921,-9.37480514412569,
2.7625273577762));
#29195=CARTESIAN_POINT('Ctrl Pts',(-2.85115657841426,-9.56992297047031,
1.17970281380798));
#29196=CARTESIAN_POINT('Ctrl Pts',(-2.84627636488886,-9.61813764156408,
0.78857830091096));
#29197=CARTESIAN_POINT('Ctrl Pts',(-2.84139615136346,-9.64186107894428,
0.394434706521363));
#29198=CARTESIAN_POINT('Ctrl Pts',(-2.83651593783807,-9.64146833476739,
0.000244149912687573));
#29199=CARTESIAN_POINT('Origin',(-3.5,0.,0.));
#29200=CARTESIAN_POINT('',(-2.08651593783807,-9.64217411726438,-0.000144835560233357));
#29201=CARTESIAN_POINT('',(-2.28848406216193,-9.64087107694564,0.000138544266770069));
#29202=CARTESIAN_POINT('',(-3.5,-9.64155,-1.18074933463192E-15));
#29203=CARTESIAN_POINT('Ctrl Pts',(-2.28848406216193,-9.64087107694564,
0.000138544266770069));
#29204=CARTESIAN_POINT('Ctrl Pts',(-2.29636870027324,-9.64119830166034,
0.637119391179249));
#29205=CARTESIAN_POINT('Ctrl Pts',(-2.30425333838455,-9.57900501984992,
1.27403718462593));
#29206=CARTESIAN_POINT('Ctrl Pts',(-2.31213797649586,-9.45365959940943,
1.89827416678697));
#29207=CARTESIAN_POINT('Ctrl Pts',(-2.3318874974108,-9.13969312845218,3.46186924382557));
#29208=CARTESIAN_POINT('Ctrl Pts',(-2.35163701832575,-8.42950549986849,
4.94590397918403));
#29209=CARTESIAN_POINT('Ctrl Pts',(-2.37138653924069,-7.40880070478383,
6.17128809492729));
#29210=CARTESIAN_POINT('Ctrl Pts',(-2.39113606015564,-6.38809590969918,
7.39667221067056));
#29211=CARTESIAN_POINT('Ctrl Pts',(-2.41088558107058,-5.05687394811357,
8.36340570679862));
#29212=CARTESIAN_POINT('Ctrl Pts',(-2.43063510198553,-3.57578396483025,
8.95482516136745));
#29213=CARTESIAN_POINT('Ctrl Pts',(-2.45038462290047,-2.09469398154692,
9.54624461593629));
#29214=CARTESIAN_POINT('Ctrl Pts',(-2.47013414381541,-0.463735976565879,
9.76235002894589));
#29215=CARTESIAN_POINT('Ctrl Pts',(-2.48988366473036,1.12026937236647,9.57706224095543));
#29216=CARTESIAN_POINT('Ctrl Pts',(-2.50963318564531,2.7042747212988,9.39177445296498));
#29217=CARTESIAN_POINT('Ctrl Pts',(-2.52938270656025,4.24132741418244,8.80509346397447));
#29218=CARTESIAN_POINT('Ctrl Pts',(-2.54913222747519,5.54593907435693,7.88781873633755));
#29219=CARTESIAN_POINT('Ctrl Pts',(-2.56888174839014,6.85055073453146,6.97054400870061));
#29220=CARTESIAN_POINT('Ctrl Pts',(-2.58863126930509,7.92272136199684,5.72267554241725));
#29221=CARTESIAN_POINT('Ctrl Pts',(-2.60838079022003,8.63306359735259,4.29480355288367));
#29222=CARTESIAN_POINT('Ctrl Pts',(-2.62813031113498,9.34340583270835,2.8669315633501));
#29223=CARTESIAN_POINT('Ctrl Pts',(-2.64787983204992,9.6919196759545,1.25905605056633));
#29224=CARTESIAN_POINT('Ctrl Pts',(-2.66762935296487,9.63654718898212,-0.334787855690263));
#29225=CARTESIAN_POINT('Ctrl Pts',(-2.68737887387981,9.58117470200974,-1.92863176194685));
#29226=CARTESIAN_POINT('Ctrl Pts',(-2.70712839479476,9.12191588481883,-3.50844406167626));
#29227=CARTESIAN_POINT('Ctrl Pts',(-2.7268779157097,8.31419315256938,-4.88357623628066));
#29228=CARTESIAN_POINT('Ctrl Pts',(-2.74662743662464,7.50647042031993,-6.25870841088505));
#29229=CARTESIAN_POINT('Ctrl Pts',(-2.76637695753959,6.35028377301195,-7.42916046036445));
#29230=CARTESIAN_POINT('Ctrl Pts',(-2.78612647845453,4.98515945155998,-8.25368462423414));
#29231=CARTESIAN_POINT('Ctrl Pts',(-2.80587599936948,3.62003513010801,-9.07820878810382));
#29232=CARTESIAN_POINT('Ctrl Pts',(-2.82562552028443,2.04597313451206,-9.55680506636378));
#29233=CARTESIAN_POINT('Ctrl Pts',(-2.84537504119937,0.452928048422888,
-9.63171743858532));
#29234=CARTESIAN_POINT('Ctrl Pts',(-2.86512456211431,-1.1401170376663,-9.70662981080687));
#29235=CARTESIAN_POINT('Ctrl Pts',(-2.88487408302926,-2.7521452142487,-9.37785827698998));
#29236=CARTESIAN_POINT('Ctrl Pts',(-2.9046236039442,-4.18862021656932,-8.68507831370239));
#29237=CARTESIAN_POINT('Ctrl Pts',(-2.92437312485915,-5.62509521888996,
-7.99229835041479));
#29238=CARTESIAN_POINT('Ctrl Pts',(-2.9441226457741,-6.8860170469488,-6.93550995765648));
#29239=CARTESIAN_POINT('Ctrl Pts',(-2.96387216668904,-7.81922023233658,
-5.64224419819056));
#29240=CARTESIAN_POINT('Ctrl Pts',(-2.98362168760399,-8.75242341772432,
-4.3489784387247));
#29241=CARTESIAN_POINT('Ctrl Pts',(-3.00337120851893,-9.35790796044102,
-2.81923531255126));
#29242=CARTESIAN_POINT('Ctrl Pts',(-3.02312072943387,-9.56260522371092,
-1.23762109276363));
#29243=CARTESIAN_POINT('Ctrl Pts',(-3.02824184034323,-9.61568384736771,
-0.827503709652114));
#29244=CARTESIAN_POINT('Ctrl Pts',(-3.03336295125258,-9.64181430822856,
-0.413898614363083));
#29245=CARTESIAN_POINT('Ctrl Pts',(-3.03848406216193,-9.6414091844932,-0.000242700028759701));
#29246=CARTESIAN_POINT('Ctrl Pts',(-2.83651593783807,-9.64146833476739,
0.000244149912687573));
#29247=CARTESIAN_POINT('Ctrl Pts',(-2.82164663044852,-9.64027169985349,
-1.20079767454136));
#29248=CARTESIAN_POINT('Ctrl Pts',(-2.80677732305897,-9.41519657160002,
-2.40227546481473));
#29249=CARTESIAN_POINT('Ctrl Pts',(-2.79190801566943,-8.9768512895793,-3.52012291183421));
#29250=CARTESIAN_POINT('Ctrl Pts',(-2.77215849475448,-8.39463793636543,
-5.00485592301334));
#29251=CARTESIAN_POINT('Ctrl Pts',(-2.75240897383954,-7.43618738395943,
-6.34205377487687));
#29252=CARTESIAN_POINT('Ctrl Pts',(-2.7326594529246,-6.21716348559042,-7.37034616439981));
#29253=CARTESIAN_POINT('Ctrl Pts',(-2.71290993200965,-4.99813958722139,
-8.39863855392276));
#29254=CARTESIAN_POINT('Ctrl Pts',(-2.6931604110947,-3.51854234288933,-9.11802548110512));
#29255=CARTESIAN_POINT('Ctrl Pts',(-2.67341089017976,-1.95692652318417,
-9.44169280227334));
#29256=CARTESIAN_POINT('Ctrl Pts',(-2.65366136926481,-0.395310703478979,
-9.76536012344156));
#29257=CARTESIAN_POINT('Ctrl Pts',(-2.63391184834987,1.24832369159934,-9.69330783859562));
#29258=CARTESIAN_POINT('Ctrl Pts',(-2.61416232743493,2.77562622346274,-9.23423107016863));
#29259=CARTESIAN_POINT('Ctrl Pts',(-2.59441280651998,4.30292875532614,-8.77515430174165));
#29260=CARTESIAN_POINT('Ctrl Pts',(-2.57466328560503,5.71389942397464,-7.92905304973361));
#29261=CARTESIAN_POINT('Ctrl Pts',(-2.55491376469009,6.83826517367314,-6.79803308348605));
#29262=CARTESIAN_POINT('Ctrl Pts',(-2.53516424377514,7.96263092337165,-5.66701311723849));
#29263=CARTESIAN_POINT('Ctrl Pts',(-2.5154147228602,8.80039175412018,-4.25107443675139));
#29264=CARTESIAN_POINT('Ctrl Pts',(-2.49566520194525,9.2504484015638,-2.72108962727205));
#29265=CARTESIAN_POINT('Ctrl Pts',(-2.47591568103031,9.70050504900742,-1.19110481779274));
#29266=CARTESIAN_POINT('Ctrl Pts',(-2.45616616011537,9.76285751314615,0.452926120678768));
#29267=CARTESIAN_POINT('Ctrl Pts',(-2.43641663920042,9.42998122607976,2.01260489550855));
#29268=CARTESIAN_POINT('Ctrl Pts',(-2.41666711828548,9.09710493901337,3.57228367033836));
#29269=CARTESIAN_POINT('Ctrl Pts',(-2.39691759737053,8.36899990074182,5.04761028152639));
#29270=CARTESIAN_POINT('Ctrl Pts',(-2.37716807645558,7.3335323387618,6.26054532975976));
#29271=CARTESIAN_POINT('Ctrl Pts',(-2.35741855554064,6.29806477678178,7.47348037799312));
#29272=CARTESIAN_POINT('Ctrl Pts',(-2.3376690346257,4.95523469109328,8.42402386327183));
#29273=CARTESIAN_POINT('Ctrl Pts',(-2.31791951371075,3.46709207118489,8.99746614106264));
#29274=CARTESIAN_POINT('Ctrl Pts',(-2.2981699927958,1.9789494512765,9.57090841885345));
#29275=CARTESIAN_POINT('Ctrl Pts',(-2.27842047188086,0.345494297148205,
9.76724948915638));
#29276=CARTESIAN_POINT('Ctrl Pts',(-2.25867095096591,-1.23615136259958,
9.56279531300263));
#29277=CARTESIAN_POINT('Ctrl Pts',(-2.23892143005097,-2.81779702234732,
9.35834113684888));
#29278=CARTESIAN_POINT('Ctrl Pts',(-2.21917190913603,-4.34763318771457,
8.75309171423847));
#29279=CARTESIAN_POINT('Ctrl Pts',(-2.19942238822108,-5.64104235782824,
7.82008730813342));
#29280=CARTESIAN_POINT('Ctrl Pts',(-2.17967286730614,-6.93445152794191,
6.88708290202836));
#29281=CARTESIAN_POINT('Ctrl Pts',(-2.15992334639119,-7.99143370280202,
5.62632351242866));
#29282=CARTESIAN_POINT('Ctrl Pts',(-2.14017382547625,-8.68443443441755,
4.18995500500241));
#29283=CARTESIAN_POINT('Ctrl Pts',(-2.12228786293019,-9.31204384243555,
2.88912176267674));
#29284=CARTESIAN_POINT('Ctrl Pts',(-2.10440190038413,-9.64112134924384,
1.44425666161893));
#29285=CARTESIAN_POINT('Ctrl Pts',(-2.08651593783807,-9.64217411726438,
-0.000144835560233357));
#29286=CARTESIAN_POINT('Origin',(-3.5,0.,0.));
#29287=CARTESIAN_POINT('',(-1.33651593783807,-9.64079438360302,-9.14169411088817E-5));
#29288=CARTESIAN_POINT('',(-1.53848406216193,-9.64228534650892,9.30951726905646E-5));
#29289=CARTESIAN_POINT('',(-3.5,-9.64155,-1.18074933463192E-15));
#29290=CARTESIAN_POINT('Ctrl Pts',(-1.53848406216193,-9.64228534650892,
9.30951726905646E-5));
#29291=CARTESIAN_POINT('Ctrl Pts',(-1.53962492837896,-9.64233187046965,
0.0922219745249846));
#29292=CARTESIAN_POINT('Ctrl Pts',(-1.54076579459598,-9.64103870036278,
0.184349545103802));
#29293=CARTESIAN_POINT('Ctrl Pts',(-1.541906660813,-9.638397502465,0.276438452957102));
#29294=CARTESIAN_POINT('Ctrl Pts',(-1.56165618172795,-9.59267575845648,
1.87058839319153));
#29295=CARTESIAN_POINT('Ctrl Pts',(-1.58140570264289,-9.1429901340128,3.45315226321777));
#29296=CARTESIAN_POINT('Ctrl Pts',(-1.60115522355784,-8.34360777096442,
4.83314949055984));
#29297=CARTESIAN_POINT('Ctrl Pts',(-1.62090474447278,-7.54422540791601,
6.21314671790196));
#29298=CARTESIAN_POINT('Ctrl Pts',(-1.64065426538773,-6.39514630626289,
7.39057730255991));
#29299=CARTESIAN_POINT('Ctrl Pts',(-1.66040378630267,-5.03503898284049,
8.22335132869036));
#29300=CARTESIAN_POINT('Ctrl Pts',(-1.68015330721762,-3.67493165941809,
9.05612535482081));
#29301=CARTESIAN_POINT('Ctrl Pts',(-1.69990282813256,-2.10379611422641,
9.54424282242376));
#29302=CARTESIAN_POINT('Ctrl Pts',(-1.71965234904751,-0.511233772864205,
9.62879871340552));
#29303=CARTESIAN_POINT('Ctrl Pts',(-1.73940186996245,1.08132856849799,9.71335460438728));
#29304=CARTESIAN_POINT('Ctrl Pts',(-1.7591513908774,2.69531770603071,9.39434891874785));
#29305=CARTESIAN_POINT('Ctrl Pts',(-1.77890091179234,4.13596073022041,8.71027861046198));
#29306=CARTESIAN_POINT('Ctrl Pts',(-1.79865043270729,5.57660375441009,8.02620830217611));
#29307=CARTESIAN_POINT('Ctrl Pts',(-1.81839995362223,6.84390066525676,6.97707337124382));
#29308=CARTESIAN_POINT('Ctrl Pts',(-1.83814947453718,7.78491666239339,5.68948127630161));
#29309=CARTESIAN_POINT('Ctrl Pts',(-1.85789899545212,8.72593265953001,4.4018891813594));
#29310=CARTESIAN_POINT('Ctrl Pts',(-1.87764851636707,9.3406677429566,2.87583992240729));
#29311=CARTESIAN_POINT('Ctrl Pts',(-1.89739803728201,9.55493693955612,1.29549400419403));
#29312=CARTESIAN_POINT('Ctrl Pts',(-1.91714755819696,9.76920613615564,-0.284851914019197));
#29313=CARTESIAN_POINT('Ctrl Pts',(-1.9368970791119,9.5830094459281,-1.91949449149356));
#29314=CARTESIAN_POINT('Ctrl Pts',(-1.95664660002685,9.01881670479375,-3.41116840380682));
#29315=CARTESIAN_POINT('Ctrl Pts',(-1.97639612094179,8.45462396365938,-4.90284231612012));
#29316=CARTESIAN_POINT('Ctrl Pts',(-1.99614564185674,7.51243517161817,-6.25154756327229));
#29317=CARTESIAN_POINT('Ctrl Pts',(-2.01589516277168,6.3059517459036,-7.29452515330038));
#29318=CARTESIAN_POINT('Ctrl Pts',(-2.03564468368663,5.09946832018903,-8.33750274332848));
#29319=CARTESIAN_POINT('Ctrl Pts',(-2.05539420460157,3.62869026080111,-9.07475267623249));
#29320=CARTESIAN_POINT('Ctrl Pts',(-2.07514372551652,2.07110805712042,-9.41730513732711));
#29321=CARTESIAN_POINT('Ctrl Pts',(-2.09489324643146,0.51352585343973,-9.75985759842174));
#29322=CARTESIAN_POINT('Ctrl Pts',(-2.11464276734641,-1.13086049453372,
-9.70771258770698));
#29323=CARTESIAN_POINT('Ctrl Pts',(-2.13439228826135,-2.66360980407379,
-9.26716285847178));
#29324=CARTESIAN_POINT('Ctrl Pts',(-2.1541418091763,-4.19635911361386,-8.82661312923658));
#29325=CARTESIAN_POINT('Ctrl Pts',(-2.17389133009124,-5.61747138472055,
-7.99765868148093));
#29326=CARTESIAN_POINT('Ctrl Pts',(-2.19364085100619,-6.7554496938074,-6.88033604326375));
#29327=CARTESIAN_POINT('Ctrl Pts',(-2.21339037192113,-7.89342800289421,
-5.7630134050466));
#29328=CARTESIAN_POINT('Ctrl Pts',(-2.23313989283608,-8.74827234996121,
-4.35732257636792));
#29329=CARTESIAN_POINT('Ctrl Pts',(-2.25288941375102,-9.21682186682932,
-2.83289945266923));
#29330=CARTESIAN_POINT('Ctrl Pts',(-2.26475429655466,-9.49831148519949,
-1.9170746190575));
#29331=CARTESIAN_POINT('Ctrl Pts',(-2.2766191793583,-9.64037866590084,-0.958396646579831));
#29332=CARTESIAN_POINT('Ctrl Pts',(-2.28848406216193,-9.64087107694564,
0.000138544266770069));
#29333=CARTESIAN_POINT('Ctrl Pts',(-2.08651593783807,-9.64217411726438,
-0.000144835560233357));
#29334=CARTESIAN_POINT('Ctrl Pts',(-2.08465237946918,-9.64228380633759,
-0.150638637119236));
#29335=CARTESIAN_POINT('Ctrl Pts',(-2.0827888211003,-9.63883252828628,-0.301127405892672));
#29336=CARTESIAN_POINT('Ctrl Pts',(-2.08092526273141,-9.63178692444962,
-0.45144770643226));
#29337=CARTESIAN_POINT('Ctrl Pts',(-2.06117574181647,-9.5571193944952,-2.04450428518778));
#29338=CARTESIAN_POINT('Ctrl Pts',(-2.04142622090152,-9.07876504621538,
-3.61863981744596));
#29339=CARTESIAN_POINT('Ctrl Pts',(-2.02167669998658,-8.25445070442347,
-4.98389084530197));
#29340=CARTESIAN_POINT('Ctrl Pts',(-2.00192717907163,-7.43013636263153,
-6.34914187315801));
#29341=CARTESIAN_POINT('Ctrl Pts',(-1.98217765815669,-6.25986202732746,
-7.50550839661188));
#29342=CARTESIAN_POINT('Ctrl Pts',(-1.96242813724174,-4.88485401281266,
-8.31344246766343));
#29343=CARTESIAN_POINT('Ctrl Pts',(-1.9426786163268,-3.50984599829794,-9.12137653871494));
#29344=CARTESIAN_POINT('Ctrl Pts',(-1.92292909541185,-1.9301043045725,-9.58087815736418));
#29345=CARTESIAN_POINT('Ctrl Pts',(-1.90317957449691,-0.336268929645929,
-9.63649560766758));
#29346=CARTESIAN_POINT('Ctrl Pts',(-1.88343005358196,1.25756644528064,-9.69211305797098));
#29347=CARTESIAN_POINT('Ctrl Pts',(-1.86368053266702,2.86549550140836,-9.34384633992854));
#29348=CARTESIAN_POINT('Ctrl Pts',(-1.84393101175207,4.29347664745853,-8.63372356908478));
#29349=CARTESIAN_POINT('Ctrl Pts',(-1.82418149083713,5.72145779350875,-7.92360079824101));
#29350=CARTESIAN_POINT('Ctrl Pts',(-1.80443196992218,6.96949102948142,-6.8516219745959));
#29351=CARTESIAN_POINT('Ctrl Pts',(-1.78468244900724,7.88696625591108,-5.54715131105702));
#29352=CARTESIAN_POINT('Ctrl Pts',(-1.76493292809229,8.80444148234076,-4.24268064751813));
#29353=CARTESIAN_POINT('Ctrl Pts',(-1.74518340717735,9.39135869922739,-2.70571814408551));
#29354=CARTESIAN_POINT('Ctrl Pts',(-1.7254338862624,9.57688993671781,-1.12174129354095));
#29355=CARTESIAN_POINT('Ctrl Pts',(-1.70568436534746,9.76242117420822,0.46223555700355));
#29356=CARTESIAN_POINT('Ctrl Pts',(-1.68593484443251,9.54656643230241,2.09322675465993));
#29357=CARTESIAN_POINT('Ctrl Pts',(-1.66618532351757,8.9553746199649,3.57440761605757));
#29358=CARTESIAN_POINT('Ctrl Pts',(-1.64643580260262,8.36418280762738,5.05558847745521));
#29359=CARTESIAN_POINT('Ctrl Pts',(-1.62668628168768,7.39765392485815,6.38695900259412));
#29360=CARTESIAN_POINT('Ctrl Pts',(-1.60693676077273,6.17242670127939,7.40785211832518));
#29361=CARTESIAN_POINT('Ctrl Pts',(-1.58718723985779,4.94719947770057,8.4287452340563));
#29362=CARTESIAN_POINT('Ctrl Pts',(-1.56743771894284,3.46327391331218,9.13916094037954));
#29363=CARTESIAN_POINT('Ctrl Pts',(-1.5476881980279,1.89972711151983,9.45336772221405));
#29364=CARTESIAN_POINT('Ctrl Pts',(-1.52793867711295,0.336180309727578,
9.76757450404853));
#29365=CARTESIAN_POINT('Ctrl Pts',(-1.50818915619801,-1.30698772946864,
9.68557236139433));
#29366=CARTESIAN_POINT('Ctrl Pts',(-1.48843963528306,-2.83148284635523,
9.21725714518358));
#29367=CARTESIAN_POINT('Ctrl Pts',(-1.46869011436812,-4.35597796324186,
8.74894192897282));
#29368=CARTESIAN_POINT('Ctrl Pts',(-1.44894059345317,-5.76180015781887,
7.89431363920549));
#29369=CARTESIAN_POINT('Ctrl Pts',(-1.42919107253823,-6.87929768167669,
6.75650707070742));
#29370=CARTESIAN_POINT('Ctrl Pts',(-1.40944155162328,-7.99679520553452,
5.61870050220935));
#29371=CARTESIAN_POINT('Ctrl Pts',(-1.38969203070834,-8.82596805867316,
4.19771565498054));
#29372=CARTESIAN_POINT('Ctrl Pts',(-1.36994250979339,-9.26675335631859,
2.66503407535437));
#29373=CARTESIAN_POINT('Ctrl Pts',(-1.35880031914162,-9.51543350628356,
1.80033308122873));
#29374=CARTESIAN_POINT('Ctrl Pts',(-1.34765812848984,-9.64049234473773,
0.90007972103179));
#29375=CARTESIAN_POINT('Ctrl Pts',(-1.33651593783807,-9.64079438360302,
-9.14169411088817E-5));
#29376=CARTESIAN_POINT('Origin',(-3.5,0.,0.));
#29377=CARTESIAN_POINT('',(-0.586515937838063,-9.64158892627347,0.000242834945830858));
#29378=CARTESIAN_POINT('',(-0.788484062161934,-9.64129453877519,-0.000235704550493598));
#29379=CARTESIAN_POINT('',(-3.5,-9.64155,-1.18074933463192E-15));
#29380=CARTESIAN_POINT('Ctrl Pts',(-0.788484062161934,-9.64129453877519,
-0.000235704550493598));
#29381=CARTESIAN_POINT('Ctrl Pts',(-0.802630677399617,-9.64022960846392,
1.14249116596726));
#29382=CARTESIAN_POINT('Ctrl Pts',(-0.816777292637301,-9.43695967827412,
2.2855868580281));
#29383=CARTESIAN_POINT('Ctrl Pts',(-0.830923907874984,-9.03930390030387,
3.35650258926584));
#29384=CARTESIAN_POINT('Ctrl Pts',(-0.850673428789929,-8.48415265231826,
4.85156499655352));
#29385=CARTESIAN_POINT('Ctrl Pts',(-0.870422949704873,-7.55014669543877,
6.20594988869364));
#29386=CARTESIAN_POINT('Ctrl Pts',(-0.890172470619819,-6.3499999590804,
7.25621286577753));
#29387=CARTESIAN_POINT('Ctrl Pts',(-0.909921991534764,-5.14985322272204,
8.30647584286142));
#29388=CARTESIAN_POINT('Ctrl Pts',(-0.929671512449711,-3.6835657068848,
9.0526169048891));
#29389=CARTESIAN_POINT('Ctrl Pts',(-0.949421033364656,-2.12808599133395,
9.40459327388937));
#29390=CARTESIAN_POINT('Ctrl Pts',(-0.969170554279602,-0.572606275783102,
9.75656964288964));
#29391=CARTESIAN_POINT('Ctrl Pts',(-0.988920075194546,1.07206563948137,
9.71438131886251));
#29392=CARTESIAN_POINT('Ctrl Pts',(-1.00866959610949,2.60745411005643,9.28311950250272));
#29393=CARTESIAN_POINT('Ctrl Pts',(-1.02841911702443,4.14284258063145,8.85185768614296));
#29394=CARTESIAN_POINT('Ctrl Pts',(-1.04816863793938,5.56894760651708,8.03152237745056));
#29395=CARTESIAN_POINT('Ctrl Pts',(-1.06791815885432,6.71366974868721,6.92110996440303));
#29396=CARTESIAN_POINT('Ctrl Pts',(-1.08766767976927,7.85839189085738,5.81069755135547));
#29397=CARTESIAN_POINT('Ctrl Pts',(-1.10741720068421,8.72173114931205,4.41020803395276));
#29398=CARTESIAN_POINT('Ctrl Pts',(-1.12716672159916,9.19950150733269,2.8886496240251));
#29399=CARTESIAN_POINT('Ctrl Pts',(-1.1469162425141,9.67727186535334,1.36709121409741));
#29400=CARTESIAN_POINT('Ctrl Pts',(-1.16666576342905,9.76947332293996,-0.275536088355169));
#29401=CARTESIAN_POINT('Ctrl Pts',(-1.186415284344,9.46497919668564,-1.84100337862394));
#29402=CARTESIAN_POINT('Ctrl Pts',(-1.20616480525894,9.16048507043134,-3.40647066889264));
#29403=CARTESIAN_POINT('Ctrl Pts',(-1.22591432617388,8.45929536033612,-4.89477794697749));
#29404=CARTESIAN_POINT('Ctrl Pts',(-1.24566384708883,7.44602820711744,-6.12631933322187));
#29405=CARTESIAN_POINT('Ctrl Pts',(-1.26541336800377,6.43276105389874,-7.3578607194663));
#29406=CARTESIAN_POINT('Ctrl Pts',(-1.28516288891872,5.10741645755655,-8.33263621387025));
#29407=CARTESIAN_POINT('Ctrl Pts',(-1.30491240983366,3.62993429447211,-8.93301190257866));
#29408=CARTESIAN_POINT('Ctrl Pts',(-1.32466193074861,2.15245213138768,-9.53338759128707));
#29409=CARTESIAN_POINT('Ctrl Pts',(-1.34441145166355,0.522832401560974,
-9.75936347429993));
#29410=CARTESIAN_POINT('Ctrl Pts',(-1.3641609725785,-1.06226571757125,-9.58366924403538));
#29411=CARTESIAN_POINT('Ctrl Pts',(-1.38391049349344,-2.64736383670343,
-9.40797501377084));
#29412=CARTESIAN_POINT('Ctrl Pts',(-1.40366001440839,-4.18794034514114,
-8.83061067022889));
#29413=CARTESIAN_POINT('Ctrl Pts',(-1.42340953532333,-5.49808161936687,
-7.92125136203724));
#29414=CARTESIAN_POINT('Ctrl Pts',(-1.44315905623828,-6.80822289359264,
-7.01189205384556));
#29415=CARTESIAN_POINT('Ctrl Pts',(-1.46290857715322,-7.88792893360642,
-5.77053778100414));
#29416=CARTESIAN_POINT('Ctrl Pts',(-1.48265809806817,-8.60690302182664,
-4.3469926393621));
#29417=CARTESIAN_POINT('Ctrl Pts',(-1.50126675276609,-9.28434429253203,
-3.00568111581648));
#29418=CARTESIAN_POINT('Ctrl Pts',(-1.51987540746401,-9.64152649476305,
-1.50261991183219));
#29419=CARTESIAN_POINT('Ctrl Pts',(-1.53848406216193,-9.64228534650892,
9.30951726905646E-5));
#29420=CARTESIAN_POINT('Ctrl Pts',(-1.33651593783807,-9.64079438360302,
-9.14169411088817E-5));
#29421=CARTESIAN_POINT('Ctrl Pts',(-1.3279086075749,-9.64102770830074,-0.695472650313908));
#29422=CARTESIAN_POINT('Ctrl Pts',(-1.31930127731173,-9.56681184096733,
-1.39080481719761));
#29423=CARTESIAN_POINT('Ctrl Pts',(-1.31069394704856,-9.41762333037316,
-2.06966064775193));
#29424=CARTESIAN_POINT('Ctrl Pts',(-1.29094442613361,-9.07531026463006,
-3.62729547920872));
#29425=CARTESIAN_POINT('Ctrl Pts',(-1.27119490521867,-8.33828639099159,
-5.09818683009872));
#29426=CARTESIAN_POINT('Ctrl Pts',(-1.25144538430372,-7.29549424377304,
-6.3048305392545));
#29427=CARTESIAN_POINT('Ctrl Pts',(-1.23169586338878,-6.25270209655455,
-7.51147424841021));
#29428=CARTESIAN_POINT('Ctrl Pts',(-1.21194634247383,-4.90414167575602,
-8.45387031583172));
#29429=CARTESIAN_POINT('Ctrl Pts',(-1.19219682155889,-3.41255449599212,
-9.01829231071637));
#29430=CARTESIAN_POINT('Ctrl Pts',(-1.17244730064394,-1.9209673162282,-9.58271430560103));
#29431=CARTESIAN_POINT('Ctrl Pts',(-1.152697779729,-0.286353377498845,-9.76916222794881));
#29432=CARTESIAN_POINT('Ctrl Pts',(-1.13294825881405,1.29402545183876,-9.55513592366089));
#29433=CARTESIAN_POINT('Ctrl Pts',(-1.11319873789911,2.87440428117639,-9.34110961937297));
#29434=CARTESIAN_POINT('Ctrl Pts',(-1.09344921698416,4.40054800112231,-8.72660908844935));
#29435=CARTESIAN_POINT('Ctrl Pts',(-1.07369969606922,5.68828470756819,-7.78579099869037));
#29436=CARTESIAN_POINT('Ctrl Pts',(-1.05395017515427,6.97602141401403,-6.84497290893142));
#29437=CARTESIAN_POINT('Ctrl Pts',(-1.03420065423933,8.02535110695982,-5.57783726033715));
#29438=CARTESIAN_POINT('Ctrl Pts',(-1.01445113332438,8.70964282428737,-4.13729939247586));
#29439=CARTESIAN_POINT('Ctrl Pts',(-0.994701612409438,9.39393454161492,
-2.69676152461457));
#29440=CARTESIAN_POINT('Ctrl Pts',(-0.974952091494494,9.71318828332421,
-1.08282143748628));
#29441=CARTESIAN_POINT('Ctrl Pts',(-0.95520257057955,9.62887716054125,0.509753878698472));
#29442=CARTESIAN_POINT('Ctrl Pts',(-0.935453049664605,9.54456603775828,
2.10232919488327));
#29443=CARTESIAN_POINT('Ctrl Pts',(-0.91570352874966,9.05669005048304,3.67353974012451));
#29444=CARTESIAN_POINT('Ctrl Pts',(-0.895954007834715,8.22412507545669,
5.03377503796996));
#29445=CARTESIAN_POINT('Ctrl Pts',(-0.876204486919769,7.39156010043033,
6.39401033581541));
#29446=CARTESIAN_POINT('Ctrl Pts',(-0.856454966004824,6.21430613765286,
7.54327038626506));
#29447=CARTESIAN_POINT('Ctrl Pts',(-0.836705445089879,4.83443178860065,
8.34286483595423));
#29448=CARTESIAN_POINT('Ctrl Pts',(-0.816955924174934,3.45455743954846,
9.14245928564339));
#29449=CARTESIAN_POINT('Ctrl Pts',(-0.797206403259989,1.87206270422148,
9.5923881345721));
#29450=CARTESIAN_POINT('Ctrl Pts',(-0.777456882345044,0.27791981206064,
9.63835488907317));
#29451=CARTESIAN_POINT('Ctrl Pts',(-0.757707361430099,-1.31622308010023,
9.68432164357423));
#29452=CARTESIAN_POINT('Ctrl Pts',(-0.737957840515153,-2.922014129095,9.32632630364767));
#29453=CARTESIAN_POINT('Ctrl Pts',(-0.718208319600208,-4.34566975397303,
8.60757101504396));
#29454=CARTESIAN_POINT('Ctrl Pts',(-0.698458798685263,-5.76932537885106,
7.88881572644025));
#29455=CARTESIAN_POINT('Ctrl Pts',(-0.678709277770318,-7.01084557961234,
6.80930048915941));
#29456=CARTESIAN_POINT('Ctrl Pts',(-0.658959756855373,-7.92040623656926,
5.49929899508776));
#29457=CARTESIAN_POINT('Ctrl Pts',(-0.639210235940428,-8.82996689352616,
4.18929750101614));
#29458=CARTESIAN_POINT('Ctrl Pts',(-0.619460715025483,-9.40756800667872,
2.64880975015375));
#29459=CARTESIAN_POINT('Ctrl Pts',(-0.599711194110539,-9.58350585451965,
1.06373865495752));
#29460=CARTESIAN_POINT('Ctrl Pts',(-0.595312775353047,-9.62268899893257,
0.71072723422002));
#29461=CARTESIAN_POINT('Ctrl Pts',(-0.590914356595555,-9.64194972140693,
0.355504488041643));
#29462=CARTESIAN_POINT('Ctrl Pts',(-0.586515937838063,-9.64158892627347,
0.000242834945830858));
#29463=CARTESIAN_POINT('Origin',(-3.5,0.,0.));
#29464=CARTESIAN_POINT('',(0.16348406216194,-9.64208031777467,-0.000174349252608778));
#29465=CARTESIAN_POINT('',(-0.0384840621619312,-9.6409393879154,0.000166496178767295));
#29466=CARTESIAN_POINT('',(-3.5,-9.64155,-1.18074933463192E-15));
#29467=CARTESIAN_POINT('Ctrl Pts',(-0.0384840621619312,-9.6409393879154,
0.000166496178767295));
#29468=CARTESIAN_POINT('Ctrl Pts',(-0.045886905505331,-9.64131207733847,
0.598212169977169));
#29469=CARTESIAN_POINT('Ctrl Pts',(-0.0532897488487309,-9.58653262653383,
1.1961904000962));
#29470=CARTESIAN_POINT('Ctrl Pts',(-0.0606925921921309,-9.47595184764967,
1.7836651068862));
#29471=CARTESIAN_POINT('Ctrl Pts',(-0.0804421131070762,-9.18094122753292,
3.35094722681577));
#29472=CARTESIAN_POINT('Ctrl Pts',(-0.100191634022022,-8.48877513866814,
4.84347249283488));
#29473=CARTESIAN_POINT('Ctrl Pts',(-0.119941154936967,-7.48298276944078,
6.08112600652889));
#29474=CARTESIAN_POINT('Ctrl Pts',(-0.139690675851912,-6.47719040021342,
7.3187795202229));
#29475=CARTESIAN_POINT('Ctrl Pts',(-0.159440196766856,-5.1577717506235,
8.30156128159181));
#29476=CARTESIAN_POINT('Ctrl Pts',(-0.179189717681801,-3.68395156600086,
8.91087119716035));
#29477=CARTESIAN_POINT('Ctrl Pts',(-0.198939238596746,-2.21013138137827,
9.52018111272887));
#29478=CARTESIAN_POINT('Ctrl Pts',(-0.218688759511691,-0.581909661722974,
9.75601918249705));
#29479=CARTESIAN_POINT('Ctrl Pts',(-0.238438280426636,1.00422312458321,
9.58992495018725));
#29480=CARTESIAN_POINT('Ctrl Pts',(-0.258187801341581,2.59035591088944,
9.42383071787745));
#29481=CARTESIAN_POINT('Ctrl Pts',(-0.277937322256526,4.13439976384655,
8.85580418348966));
#29482=CARTESIAN_POINT('Ctrl Pts',(-0.297686843171471,5.45002262786544,
7.95439362801577));
#29483=CARTESIAN_POINT('Ctrl Pts',(-0.317436364086416,6.76564549188433,
7.05298307254187));
#29484=CARTESIAN_POINT('Ctrl Pts',(-0.337185885001362,7.85284736696499,
5.81818849598189));
#29485=CARTESIAN_POINT('Ctrl Pts',(-0.356935405916307,8.58042695348651,
4.39902238340523));
#29486=CARTESIAN_POINT('Ctrl Pts',(-0.376684926831252,9.308006540008,2.97985627082861));
#29487=CARTESIAN_POINT('Ctrl Pts',(-0.396434447746196,9.67596383797037,
1.37631862223533));
#29488=CARTESIAN_POINT('Ctrl Pts',(-0.41618396866114,9.63989451289301,-0.218078917157266));
#29489=CARTESIAN_POINT('Ctrl Pts',(-0.435933489576085,9.60382518781565,
-1.81247645654993));
#29490=CARTESIAN_POINT('Ctrl Pts',(-0.455683010491032,9.16372923969851,
-3.39773388674197));
#29491=CARTESIAN_POINT('Ctrl Pts',(-0.475432531405977,8.37271654784118,
-4.78254558193465));
#29492=CARTESIAN_POINT('Ctrl Pts',(-0.495182052320922,7.58170385598388,
-6.16735727712726));
#29493=CARTESIAN_POINT('Ctrl Pts',(-0.514931573235866,6.43977442038642,
-7.35172323732058));
#29494=CARTESIAN_POINT('Ctrl Pts',(-0.534681094150811,5.08473395079955,
-8.19271659972427));
#29495=CARTESIAN_POINT('Ctrl Pts',(-0.554430615065756,3.72969348121264,
-9.03370996212798));
#29496=CARTESIAN_POINT('Ctrl Pts',(-0.574180135980702,2.16154197763633,
-9.53133072674204));
#29497=CARTESIAN_POINT('Ctrl Pts',(-0.593929656895646,0.569520757628604,
-9.62552703702085));
#29498=CARTESIAN_POINT('Ctrl Pts',(-0.613679177810591,-1.02250046237912,
-9.71972334729966));
#29499=CARTESIAN_POINT('Ctrl Pts',(-0.633428698725536,-2.63839139881825,
-9.41049520324323));
#29500=CARTESIAN_POINT('Ctrl Pts',(-0.653178219640481,-4.08314963697168,
-8.73515962509546));
#29501=CARTESIAN_POINT('Ctrl Pts',(-0.672927740555426,-5.52790787512507,
-8.05982404694771));
#29502=CARTESIAN_POINT('Ctrl Pts',(-0.692677261470371,-6.80153341499276,
-7.01838103470866));
#29503=CARTESIAN_POINT('Ctrl Pts',(-0.712426782385315,-7.75032773019536,
-5.73650980199293));
#29504=CARTESIAN_POINT('Ctrl Pts',(-0.73217630330026,-8.69912204539795,
-4.45463856927719));
#29505=CARTESIAN_POINT('Ctrl Pts',(-0.751925824215204,-9.32308513593545,
-2.93233911608478));
#29506=CARTESIAN_POINT('Ctrl Pts',(-0.771675345130148,-9.54691841165834,
-1.35331942827096));
#29507=CARTESIAN_POINT('Ctrl Pts',(-0.77727825080741,-9.61041953336701,
-0.905354213749452));
#29508=CARTESIAN_POINT('Ctrl Pts',(-0.782881156484672,-9.64171631486697,
-0.452823886444953));
#29509=CARTESIAN_POINT('Ctrl Pts',(-0.788484062161934,-9.64129453877519,
-0.000235704550493598));
#29510=CARTESIAN_POINT('Ctrl Pts',(-0.586515937838063,-9.64158892627347,
0.000242834945830858));
#29511=CARTESIAN_POINT('Ctrl Pts',(-0.57116483568061,-9.64032970034318,
-1.2396704679906));
#29512=CARTESIAN_POINT('Ctrl Pts',(-0.555813733523157,-9.40005910021102,
-2.48005769939615));
#29513=CARTESIAN_POINT('Ctrl Pts',(-0.540462631365704,-8.93356968403343,
-3.62856129754286));
#29514=CARTESIAN_POINT('Ctrl Pts',(-0.52071311045076,-8.333421083177,-5.10613571531682));
#29515=CARTESIAN_POINT('Ctrl Pts',(-0.500963589535815,-7.35884929893488,
-6.43163011133468));
#29516=CARTESIAN_POINT('Ctrl Pts',(-0.481214068620871,-6.1274636618099,
-7.4450865316139));
#29517=CARTESIAN_POINT('Ctrl Pts',(-0.461464547705925,-4.89607802468489,
-8.45854295189315));
#29518=CARTESIAN_POINT('Ctrl Pts',(-0.44171502679098,-3.40787853467704,
-9.15996139643373));
#29519=CARTESIAN_POINT('Ctrl Pts',(-0.421965505876035,-1.84245806384899,
-9.46469612147266));
#29520=CARTESIAN_POINT('Ctrl Pts',(-0.402215984961089,-0.277037593020945,
-9.76943084651159));
#29521=CARTESIAN_POINT('Ctrl Pts',(-0.382466464046144,1.36560385862727,
-9.67748185204887));
#29522=CARTESIAN_POINT('Ctrl Pts',(-0.362716943131199,2.88723567898901,
-9.19994535444941));
#29523=CARTESIAN_POINT('Ctrl Pts',(-0.342967422216254,4.40886749935072,
-8.72240885684995));
#29524=CARTESIAN_POINT('Ctrl Pts',(-0.32321790130131,5.80948968842594,-7.85928485611378));
#29525=CARTESIAN_POINT('Ctrl Pts',(-0.303468380386366,6.92007802364878,
-6.71473339269328));
#29526=CARTESIAN_POINT('Ctrl Pts',(-0.283718859471421,8.03066635887166,
-5.57018192927274));
#29527=CARTESIAN_POINT('Ctrl Pts',(-0.263969338556473,8.85122084024217,
-4.14420300316775));
#29528=CARTESIAN_POINT('Ctrl Pts',(-0.244219817641528,9.28271863083791,
-2.60888083479162));
#29529=CARTESIAN_POINT('Ctrl Pts',(-0.224470296726584,9.71421642143363,
-1.07355866641553));
#29530=CARTESIAN_POINT('Ctrl Pts',(-0.204720775811639,9.75665752125467,
0.571106744231792));
#29531=CARTESIAN_POINT('Ctrl Pts',(-0.184971254896695,9.40492022443375,
2.12664053549246));
#29532=CARTESIAN_POINT('Ctrl Pts',(-0.16522173398175,9.05318292761283,3.68217432675312));
#29533=CARTESIAN_POINT('Ctrl Pts',(-0.145472213066806,8.30726723414997,
5.1485764986271));
#29534=CARTESIAN_POINT('Ctrl Pts',(-0.125722692151861,7.25718872636263,
6.34888463917673));
#29535=CARTESIAN_POINT('Ctrl Pts',(-0.105973171236915,6.20711021857523,
7.54919277972643));
#29536=CARTESIAN_POINT('Ctrl Pts',(-0.0862236503219702,4.85286889646334,
8.48340688895172));
#29537=CARTESIAN_POINT('Ctrl Pts',(-0.0664741294070245,3.35789183156476,
9.03878790976793));
#29538=CARTESIAN_POINT('Ctrl Pts',(-0.0467246084920799,1.86291476666626,
9.5941689305841));
#29539=CARTESIAN_POINT('Ctrl Pts',(-0.0269750875771353,0.22720195898112,
9.77071686299123));
#29540=CARTESIAN_POINT('Ctrl Pts',(-0.00722556666219065,-1.35185210879035,
9.54712627940369));
#29541=CARTESIAN_POINT('Ctrl Pts',(0.0125239542527545,-2.93090617656187,
9.32353569581614));
#29542=CARTESIAN_POINT('Ctrl Pts',(0.0322734751676994,-4.45330150441969,
8.69980659623389));
#29543=CARTESIAN_POINT('Ctrl Pts',(0.0520229960826446,-5.73531854636519,
7.75120930243113));
#29544=CARTESIAN_POINT('Ctrl Pts',(0.0717725169975898,-7.01733558831068,
6.80261200862837));
#29545=CARTESIAN_POINT('Ctrl Pts',(0.0915220379125351,-8.05897434434382,
5.52914652060512));
#29546=CARTESIAN_POINT('Ctrl Pts',(0.11127155882748,-8.73453195993958,4.08449210952313));
#29547=CARTESIAN_POINT('Ctrl Pts',(0.128675726605634,-9.32986377260853,
2.81139754382694));
#29548=CARTESIAN_POINT('Ctrl Pts',(0.146079894383787,-9.64089958585323,
1.40535888296871));
#29549=CARTESIAN_POINT('Ctrl Pts',(0.16348406216194,-9.64208031777467,-0.000174349252608778));
#29550=CARTESIAN_POINT('Origin',(-3.5,0.,0.));
#29551=CARTESIAN_POINT('',(0.913484062161936,-9.64080718149228,-0.000193112876372633));
#29552=CARTESIAN_POINT('',(0.711515937838069,-9.64233463315361,5.55577575209881E-5));
#29553=CARTESIAN_POINT('',(-3.5,-9.64155,-1.18074933463192E-15));
#29554=CARTESIAN_POINT('',(1.,-7.21801009705401,-6.39216838336776));
#29555=CARTESIAN_POINT('Ctrl Pts',(0.913484062161936,-9.64080718149228,
-0.000193112876372633));
#29556=CARTESIAN_POINT('Ctrl Pts',(0.922573187193013,-9.64097580048578,
-0.734553316280234));
#29557=CARTESIAN_POINT('Ctrl Pts',(0.93166231222409,-9.55814059309284,-1.46884207590725));
#29558=CARTESIAN_POINT('Ctrl Pts',(0.940751437255168,-9.39189433566671,
-2.18363780626507));
#29559=CARTESIAN_POINT('Ctrl Pts',(0.960500958170112,-9.03066221190976,
-3.73679866370149));
#29560=CARTESIAN_POINT('Ctrl Pts',(0.980250479085056,-8.27561480792393,
-5.1979255186751));
#29561=CARTESIAN_POINT('Ctrl Pts',(1.,-7.21801009705401,-6.39216838336776));
#29562=CARTESIAN_POINT('',(0.999999999999999,7.21857426272793,-6.39248696093098));
#29563=CARTESIAN_POINT('Origin',(1.,0.,0.));
#29564=CARTESIAN_POINT('Ctrl Pts',(0.999999999999999,7.21857426272793,-6.39248696093098));
#29565=CARTESIAN_POINT('Ctrl Pts',(0.982177658156687,6.26356489870851,-7.46927130190886));
#29566=CARTESIAN_POINT('Ctrl Pts',(0.964355316313374,5.06448313860702,-8.33050693920671));
#29567=CARTESIAN_POINT('Ctrl Pts',(0.946532974470062,3.73783082533989,-8.88839338664454));
#29568=CARTESIAN_POINT('Ctrl Pts',(0.926783453555117,2.26772393152777,-9.50660563724011));
#29569=CARTESIAN_POINT('Ctrl Pts',(0.907033932640172,0.640965728191514,
-9.75231775629702));
#29570=CARTESIAN_POINT('Ctrl Pts',(0.887284411725227,-0.946142180621593,
-9.59583455469918));
#29571=CARTESIAN_POINT('Ctrl Pts',(0.867534890810282,-2.5332500894347,-9.43935135310134));
#29572=CARTESIAN_POINT('Ctrl Pts',(0.847785369895337,-4.08070770372466,
-8.88067283084875));
#29573=CARTESIAN_POINT('Ctrl Pts',(0.828035848980391,-5.40176465919483,
-7.98724151005226));
#29574=CARTESIAN_POINT('Ctrl Pts',(0.808286328065446,-6.72282161466503,
-7.09381018925575));
#29575=CARTESIAN_POINT('Ctrl Pts',(0.7885368071505,-7.81747791131544,-5.86562606991532));
#29576=CARTESIAN_POINT('Ctrl Pts',(0.768787286235554,-8.55363594974757,
-4.45089233265519));
#29577=CARTESIAN_POINT('Ctrl Pts',(0.749696836769726,-9.26522727857401,
-3.08337040465096));
#29578=CARTESIAN_POINT('Ctrl Pts',(0.730606387303897,-9.64184836527695,
-1.54154199328144));
#29579=CARTESIAN_POINT('Ctrl Pts',(0.711515937838069,-9.64233463315361,
5.55577575209881E-5));
#29580=CARTESIAN_POINT('Origin',(-9.65625985035617,0.,0.));
#29581=CARTESIAN_POINT('',(0.406259850356178,-10.0626034466932,-0.000181953202540996));
#29582=CARTESIAN_POINT('',(0.468740149643834,-10.06286885361,5.79808157464514E-5));
#29583=CARTESIAN_POINT('',(-9.65625985035617,-10.06205,-4.69647557663214E-13));
#29584=CARTESIAN_POINT('',(1.,2.60344811511698,9.71940883564396));
#29585=CARTESIAN_POINT('Ctrl Pts',(0.468740149643834,-10.06286885361,5.79808157466586E-5));
#29586=CARTESIAN_POINT('Ctrl Pts',(0.487830599109663,-10.0623613779771,
-1.60877375665718));
#29587=CARTESIAN_POINT('Ctrl Pts',(0.526670569490437,-9.26269841475242,
-4.88247010492393));
#29588=CARTESIAN_POINT('Ctrl Pts',(0.585260060786157,-5.87362828986304,
-8.68494410471449));
#29589=CARTESIAN_POINT('Ctrl Pts',(0.644508623530991,-1.02878615726,-10.4340771460299));
#29590=CARTESIAN_POINT('Ctrl Pts',(0.703757186275826,4.0643334282463,-9.66479182544668));
#29591=CARTESIAN_POINT('Ctrl Pts',(0.763005749020661,8.1765526549945,-6.56302991227287));
#29592=CARTESIAN_POINT('Ctrl Pts',(0.822254311765496,10.3152148975558,-1.8768974633799));
#29593=CARTESIAN_POINT('Ctrl Pts',(0.88150287451033,9.96442833619652,3.26156383705692));
#29594=CARTESIAN_POINT('Ctrl Pts',(0.940751437255166,7.20829597612923,7.61418408655239));
#29595=CARTESIAN_POINT('Ctrl Pts',(0.980250479085055,4.21155540437341,9.28866001522528));
#29596=CARTESIAN_POINT('Ctrl Pts',(1.,2.60344811511698,9.71940883564396));
#29597=CARTESIAN_POINT('',(0.999999999999999,-2.60375578640692,9.7200109471421));
#29598=CARTESIAN_POINT('Origin',(1.,0.,0.));
#29599=CARTESIAN_POINT('Ctrl Pts',(0.406259850356178,-10.0626034466932,
-0.000181953202541413));
#29600=CARTESIAN_POINT('Ctrl Pts',(0.408605203492968,-10.0627694993772,
-0.197849655297783));
#29601=CARTESIAN_POINT('Ctrl Pts',(0.430700077544703,-10.0090126457275,
-2.05992802286849));
#29602=CARTESIAN_POINT('Ctrl Pts',(0.472544472511383,-8.90922609310004,
-5.52753257240065));
#29603=CARTESIAN_POINT('Ctrl Pts',(0.531793035256219,-5.20171515149495,
-9.10330010082978));
#29604=CARTESIAN_POINT('Ctrl Pts',(0.591041598001052,-0.23874007198555,
-10.4819341046316));
#29605=CARTESIAN_POINT('Ctrl Pts',(0.650290160745889,4.78185742115312,-9.33068794050316));
#29606=CARTESIAN_POINT('Ctrl Pts',(0.709538723490722,8.64832326230869,-5.92743167035388));
#29607=CARTESIAN_POINT('Ctrl Pts',(0.768787286235557,10.4274692096169,-1.09354201610874));
#29608=CARTESIAN_POINT('Ctrl Pts',(0.828035848980392,9.68987600895932,4.00425592589309));
#29609=CARTESIAN_POINT('Ctrl Pts',(0.887284411725228,6.61358904227201,8.1356504120078));
#29610=CARTESIAN_POINT('Ctrl Pts',(0.94460579539843,2.09302808608892,10.2328567692711));
#29611=CARTESIAN_POINT('Ctrl Pts',(0.982177658156686,-1.15257241662438,
10.1075740191406));
#29612=CARTESIAN_POINT('Ctrl Pts',(0.999999999999999,-2.60375578640692,
9.7200109471421));
#29613=CARTESIAN_POINT('Origin',(-9.65625985035617,0.,0.));
#29614=CARTESIAN_POINT('',(-0.343740149643824,-10.0620906239775,0.00025342578346299));
#29615=CARTESIAN_POINT('',(-0.281259850356166,-10.0614127570955,0.000173757629795403));
#29616=CARTESIAN_POINT('',(-9.65625985035617,-10.06205,-4.69647557663214E-13));
#29617=CARTESIAN_POINT('Ctrl Pts',(-0.281259850356166,-10.0614127570955,
0.000173757629795546));
#29618=CARTESIAN_POINT('Ctrl Pts',(-0.268913172784621,-10.0607640655635,
-1.04076580315036));
#29619=CARTESIAN_POINT('Ctrl Pts',(-0.236816974298132,-9.64287151587488,
-3.74728231997338));
#29620=CARTESIAN_POINT('Ctrl Pts',(-0.184971254896697,-7.25443294882962,
-7.56975066843671));
#29621=CARTESIAN_POINT('Ctrl Pts',(-0.125722692151862,-2.7740584993699,
-10.1110099362393));
#29622=CARTESIAN_POINT('Ctrl Pts',(-0.0664741294070278,2.37585137208773,
-10.211917205029));
#29623=CARTESIAN_POINT('Ctrl Pts',(-0.00722556666219231,6.95233546092519,
-7.848117856984));
#29624=CARTESIAN_POINT('Ctrl Pts',(0.0520229960826416,9.85083230810637,
-3.59012893818949));
#29625=CARTESIAN_POINT('Ctrl Pts',(0.111271558827477,10.3717725107696,1.53435894975116));
#29626=CARTESIAN_POINT('Ctrl Pts',(0.170520121572311,8.38942417794793,6.28851998843207));
#29627=CARTESIAN_POINT('Ctrl Pts',(0.229768684317148,4.38223859253949,9.52491003146027));
#29628=CARTESIAN_POINT('Ctrl Pts',(0.289017247061982,-0.682625920371043,
10.4624058141013));
#29629=CARTESIAN_POINT('Ctrl Pts',(0.348265809806817,-5.58273513680522,
8.8747398847227));
#29630=CARTESIAN_POINT('Ctrl Pts',(0.407514372551651,-9.13541725268214,
5.14509959176606));
#29631=CARTESIAN_POINT('Ctrl Pts',(0.447672485830657,-10.0489412906938,
1.7755089194844));
#29632=CARTESIAN_POINT('Ctrl Pts',(0.468081078194718,-10.0628863735066,
0.0556006785662035));
#29633=CARTESIAN_POINT('Ctrl Pts',(0.468740149643834,-10.06286885361,5.79808157466586E-5));
#29634=CARTESIAN_POINT('Ctrl Pts',(-0.343740149643824,-10.0620906239775,
0.000253425783462886));
#29635=CARTESIAN_POINT('Ctrl Pts',(-0.328389047486372,-10.0607764790244,
-1.29373661210569));
#29636=CARTESIAN_POINT('Ctrl Pts',(-0.293288424413976,-9.48743216442293,
-4.25360338997758));
#29637=CARTESIAN_POINT('Ctrl Pts',(-0.238438280426636,-6.66271704930368,
-8.09543845639));
#29638=CARTESIAN_POINT('Ctrl Pts',(-0.1791897176818,-2.00340262005729,-10.2914673500501));
#29639=CARTESIAN_POINT('Ctrl Pts',(-0.119941154936964,3.13944487393184,
-10.0035897640602));
#29640=CARTESIAN_POINT('Ctrl Pts',(-0.0606925921921299,7.52456878997794,
-7.3012866535828));
#29641=CARTESIAN_POINT('Ctrl Pts',(-0.00144402944729414,10.0935935482191,
-2.83677485203218));
#29642=CARTESIAN_POINT('Ctrl Pts',(0.0578045332975393,10.2264698394132,
2.3124093336654));
#29643=CARTESIAN_POINT('Ctrl Pts',(0.117053096042374,7.89112718079254,6.90347984831441));
#29644=CARTESIAN_POINT('Ctrl Pts',(0.176301658787208,3.65121433633638,9.82835471108965));
#29645=CARTESIAN_POINT('Ctrl Pts',(0.235550221532044,-1.46994068227644,
10.3810980324261));
#29646=CARTESIAN_POINT('Ctrl Pts',(0.294798784276879,-6.23631680707128,
8.42830204429616));
#29647=CARTESIAN_POINT('Ctrl Pts',(0.351701993884924,-9.36842634388113,
4.59911138032189));
#29648=CARTESIAN_POINT('Ctrl Pts',(0.388855682578024,-10.0613712191333,
1.46665124885246));
#29649=CARTESIAN_POINT('Ctrl Pts',(0.406259850356178,-10.0626034466932,
-0.000181953202541413));
#29650=CARTESIAN_POINT('Origin',(-9.65625985035617,0.,0.));
#29651=CARTESIAN_POINT('',(-1.09374014964383,-10.0612614286637,-9.54039379347238E-5));
#29652=CARTESIAN_POINT('',(-1.03125985035617,-10.0617833972632,-0.000245984408346792));
#29653=CARTESIAN_POINT('',(-9.65625985035617,-10.06205,-4.69647557663214E-13));
#29654=CARTESIAN_POINT('Ctrl Pts',(-1.03125985035617,-10.0617833972632,
-0.000245984408347166));
#29655=CARTESIAN_POINT('Ctrl Pts',(-1.02565694467891,-10.0622235684104,
-0.472573039252344));
#29656=CARTESIAN_POINT('Ctrl Pts',(-1.0003045180867,-9.91443341033051,-2.60951892962658));
#29657=CARTESIAN_POINT('Ctrl Pts',(-0.955202570579548,-8.42734344184841,
-6.23761212968768));
#29658=CARTESIAN_POINT('Ctrl Pts',(-0.895954007834717,-4.43982570971225,
-9.49820352670374));
#29659=CARTESIAN_POINT('Ctrl Pts',(-0.836705445089881,0.619270202354978,
-10.4663473563483));
#29660=CARTESIAN_POINT('Ctrl Pts',(-0.777456882345046,5.52890159042847,
-8.90837638241207));
#29661=CARTESIAN_POINT('Ctrl Pts',(-0.71820831960021,9.10409989696232,-5.20031610898184));
#29662=CARTESIAN_POINT('Ctrl Pts',(-0.658959756855376,10.4819698768157,
-0.237128802336295));
#29663=CARTESIAN_POINT('Ctrl Pts',(-0.599711194110542,9.32995446540496,
4.78329094252682));
#29664=CARTESIAN_POINT('Ctrl Pts',(-0.540462631365705,5.92609939215782,
8.64923514311966));
#29665=CARTESIAN_POINT('Ctrl Pts',(-0.481214068620872,1.09194519994383,
10.4276353143587));
#29666=CARTESIAN_POINT('Ctrl Pts',(-0.421965505876034,-4.0057564209339,
9.68926406183886));
#29667=CARTESIAN_POINT('Ctrl Pts',(-0.362716943131203,-8.13664505080342,
6.61233165305132));
#29668=CARTESIAN_POINT('Ctrl Pts',(-0.315815057957911,-9.85211717613616,
2.9132404502305));
#29669=CARTESIAN_POINT('Ctrl Pts',(-0.288662693699566,-10.0618017007414,
0.624302188436377));
#29670=CARTESIAN_POINT('Ctrl Pts',(-0.281259850356166,-10.0614127570955,
0.000173757629795546));
#29671=CARTESIAN_POINT('Ctrl Pts',(-1.09374014964383,-10.0612614286637,
-9.54039379352789E-5));
#29672=CARTESIAN_POINT('Ctrl Pts',(-1.08513281938066,-10.061504929426,-0.725804521170841));
#29673=CARTESIAN_POINT('Ctrl Pts',(-1.05677596820255,-9.80633710117914,
-3.11648464536511));
#29674=CARTESIAN_POINT('Ctrl Pts',(-1.00866959610949,-7.93277880763296,
-6.85557748609057));
#29675=CARTESIAN_POINT('Ctrl Pts',(-0.949421033364655,-3.7106519560076,
-9.80606875052385));
#29676=CARTESIAN_POINT('Ctrl Pts',(-0.890172470619817,1.40706267976922,
-10.3898073559533));
#29677=CARTESIAN_POINT('Ctrl Pts',(-0.830923907874984,6.18517442029282,
-8.46590453933774));
#29678=CARTESIAN_POINT('Ctrl Pts',(-0.771675345130147,9.47045775240396,
-4.49870561812545));
#29679=CARTESIAN_POINT('Ctrl Pts',(-0.712426782385315,10.4699901237859,
0.554282496966878));
#29680=CARTESIAN_POINT('Ctrl Pts',(-0.65317821964048,8.94252848812691,5.47349125491902));
#29681=CARTESIAN_POINT('Ctrl Pts',(-0.593929656895644,5.25673474038977,
9.07164054335094));
#29682=CARTESIAN_POINT('Ctrl Pts',(-0.53468109415081,0.302196989220137,
10.4802957619713));
#29683=CARTESIAN_POINT('Ctrl Pts',(-0.475432531405974,-4.72527779166189,
9.35946964684205));
#29684=CARTESIAN_POINT('Ctrl Pts',(-0.41618396866114,-8.61227884524871,
5.97968020636365));
#29685=CARTESIAN_POINT('Ctrl Pts',(-0.372286508073756,-9.95211121964369,
2.40628792237205));
#29686=CARTESIAN_POINT('Ctrl Pts',(-0.348138568401317,-10.0624671545843,
0.371009218838945));
#29687=CARTESIAN_POINT('Ctrl Pts',(-0.343740149643824,-10.0620906239775,
0.000253425783462886));
#29688=CARTESIAN_POINT('Origin',(-9.65625985035617,0.,0.));
#29689=CARTESIAN_POINT('',(-1.84374014964383,-10.06270133709,-0.000151152320359005));
#29690=CARTESIAN_POINT('',(-1.78125985035617,-10.0628174174111,9.71553621948886E-5));
#29691=CARTESIAN_POINT('',(-9.65625985035617,-10.06205,-4.69647557663214E-13));
#29692=CARTESIAN_POINT('Ctrl Pts',(-1.78125985035617,-10.0628174174111,
9.71553621948243E-5));
#29693=CARTESIAN_POINT('Ctrl Pts',(-1.76265119565825,-10.0620254696216,
-1.56815415403654));
#29694=CARTESIAN_POINT('Ctrl Pts',(-1.72429302004538,-9.2936519492452,-4.80155274286011));
#29695=CARTESIAN_POINT('Ctrl Pts',(-1.66618532351757,-5.97835648900369,
-8.61319779510975));
#29696=CARTESIAN_POINT('Ctrl Pts',(-1.60693676077273,-1.15505799756011,
-10.4208331523717));
#29697=CARTESIAN_POINT('Ctrl Pts',(-1.5476881980279,3.94702056942422,-9.71333882822164));
#29698=CARTESIAN_POINT('Ctrl Pts',(-1.48843963528306,8.0964623901765,-6.66147275996483));
#29699=CARTESIAN_POINT('Ctrl Pts',(-1.42919107253823,10.2917751528953,-2.00182086349988));
#29700=CARTESIAN_POINT('Ctrl Pts',(-1.36994250979339,10.0031071452691,3.14098233162225));
#29701=CARTESIAN_POINT('Ctrl Pts',(-1.31069394704856,7.30013009732543,7.52569087389453));
#29702=CARTESIAN_POINT('Ctrl Pts',(-1.25144538430372,2.83522349754239,10.0940294375576));
#29703=CARTESIAN_POINT('Ctrl Pts',(-1.19219682155889,-2.31398105307032,
10.2261143281957));
#29704=CARTESIAN_POINT('Ctrl Pts',(-1.13294825881405,-6.90469259801799,
7.89006607666695));
#29705=CARTESIAN_POINT('Ctrl Pts',(-1.07930260174648,-9.55238338000605,
4.05069827845285));
#29706=CARTESIAN_POINT('Ctrl Pts',(-1.04540646559385,-10.0606720218061,
1.19231899814043));
#29707=CARTESIAN_POINT('Ctrl Pts',(-1.03125985035617,-10.0617833972632,
-0.000245984408347166));
#29708=CARTESIAN_POINT('Ctrl Pts',(-1.84374014964383,-10.06270133709,-0.000151152320359421));
#29709=CARTESIAN_POINT('Ctrl Pts',(-1.84187659127494,-10.0628158100678,
-0.157208488119574));
#29710=CARTESIAN_POINT('Ctrl Pts',(-1.82026351199111,-10.0210430463493,
-1.97865888614579));
#29711=CARTESIAN_POINT('Ctrl Pts',(-1.77890091179234,-8.97550315697813,
-5.41924951978578));
#29712=CARTESIAN_POINT('Ctrl Pts',(-1.71965234904751,-5.31156150582896,
-9.03964803786181));
#29713=CARTESIAN_POINT('Ctrl Pts',(-1.66040378630267,-0.365643087312114,
-10.4782740664349));
#29714=CARTESIAN_POINT('Ctrl Pts',(-1.60115522355784,4.66852545173299,-9.38790670943975));
#29715=CARTESIAN_POINT('Ctrl Pts',(-1.541906660813,8.57591777620947,-6.03171257391441));
#29716=CARTESIAN_POINT('Ctrl Pts',(-1.48265809806816,10.4134616510556,-1.2197289537503));
#29717=CARTESIAN_POINT('Ctrl Pts',(-1.42340953532333,9.73765499990719,3.88664345951686));
#29718=CARTESIAN_POINT('Ctrl Pts',(-1.3641609725785,6.71160775287686,8.05495149893194));
#29719=CARTESIAN_POINT('Ctrl Pts',(-1.30491240983366,2.06567430073889,10.2791493792964));
#29720=CARTESIAN_POINT('Ctrl Pts',(-1.24566384708883,-3.07882185458713,
10.022413794408));
#29721=CARTESIAN_POINT('Ctrl Pts',(-1.18641528434399,-7.48022615564147,
7.34670939530617));
#29722=CARTESIAN_POINT('Ctrl Pts',(-1.13577405186233,-9.69909887236656,
3.54414338453905));
#29723=CARTESIAN_POINT('Ctrl Pts',(-1.1048823402956,-10.060946216881,0.939335185421873));
#29724=CARTESIAN_POINT('Ctrl Pts',(-1.09374014964383,-10.0612614286637,
-9.54039379352789E-5));
#29725=CARTESIAN_POINT('Origin',(-9.65625985035617,0.,0.));
#29726=CARTESIAN_POINT('',(-2.59374014964383,-10.0619647730755,0.000254798100391557));
#29727=CARTESIAN_POINT('',(-2.53125985035617,-10.0613414668576,0.000144586642133095));
#29728=CARTESIAN_POINT('',(-9.65625985035617,-10.06205,-4.69647557663214E-13));
#29729=CARTESIAN_POINT('Ctrl Pts',(-2.53125985035617,-10.0613414668576,
0.000144586642132558));
#29730=CARTESIAN_POINT('Ctrl Pts',(-2.51939496755253,-10.0608275801326,
-1.0001955056727));
#29731=CARTESIAN_POINT('Ctrl Pts',(-2.48778056383395,-9.66577498641524,
-3.6660344256632));
#29732=CARTESIAN_POINT('Ctrl Pts',(-2.43641663920042,-7.34555965317983,
-7.48135522140693));
#29733=CARTESIAN_POINT('Ctrl Pts',(-2.37716807645559,-2.8962845695608,-10.0766789300553));
#29734=CARTESIAN_POINT('Ctrl Pts',(-2.31791951371075,2.25202591556642,-10.2399366132273));
#29735=CARTESIAN_POINT('Ctrl Pts',(-2.25867095096592,6.85679663369709,-7.93172506403346));
#29736=CARTESIAN_POINT('Ctrl Pts',(-2.19942238822108,9.80663895208724,-3.70914478427321));
#29737=CARTESIAN_POINT('Ctrl Pts',(-2.14017382547625,10.3895909899559,1.40865951483102));
#29738=CARTESIAN_POINT('Ctrl Pts',(-2.08092526273141,8.46495382699166,6.18647551310075));
#29739=CARTESIAN_POINT('Ctrl Pts',(-2.02167669998658,4.49725001947583,9.47114907651764));
#29740=CARTESIAN_POINT('Ctrl Pts',(-1.96242813724174,-0.555891664582547,
10.4699048240442));
#29741=CARTESIAN_POINT('Ctrl Pts',(-1.90317957449691,-5.47486560938269,
8.941687152126));
#29742=CARTESIAN_POINT('Ctrl Pts',(-1.84393101175207,-9.072448376092,5.25534042954797));
#29743=CARTESIAN_POINT('Ctrl Pts',(-1.80329110370516,-10.0381540192056,
1.85676423142571));
#29744=CARTESIAN_POINT('Ctrl Pts',(-1.78240071657319,-10.0628659704362,
0.0962440809588831));
#29745=CARTESIAN_POINT('Ctrl Pts',(-1.78125985035617,-10.0628174174111,
9.71553621948243E-5));
#29746=CARTESIAN_POINT('Ctrl Pts',(-2.59374014964383,-10.0619647730755,
0.000254798100391383));
#29747=CARTESIAN_POINT('Ctrl Pts',(-2.57887084225428,-10.0607159489408,
-1.25316844709838));
#29748=CARTESIAN_POINT('Ctrl Pts',(-2.54425201394979,-9.51384009969817,
-4.1724567398586));
#29749=CARTESIAN_POINT('Ctrl Pts',(-2.48988366473036,-6.76025243720484,
-8.01416928096036));
#29750=CARTESIAN_POINT('Ctrl Pts',(-2.43063510198552,-2.12787026245138,
-10.2664546180655));
#29751=CARTESIAN_POINT('Ctrl Pts',(-2.37138653924069,3.01808597850499,-10.0408704455826));
#29752=CARTESIAN_POINT('Ctrl Pts',(-2.31213797649586,7.43560932790665,-7.39186283702356));
#29753=CARTESIAN_POINT('Ctrl Pts',(-2.25288941375102,10.0585044123173,-2.95878543764436));
#29754=CARTESIAN_POINT('Ctrl Pts',(-2.19364085100618,10.2537199985417,2.18841231721289));
#29755=CARTESIAN_POINT('Ctrl Pts',(-2.13439228826135,7.97413965087761,6.80742382307171));
#29756=CARTESIAN_POINT('Ctrl Pts',(-2.07514372551652,3.76995356138932,9.78342334888923));
#29757=CARTESIAN_POINT('Ctrl Pts',(-2.01589516277168,-1.34413310525547,
10.3981358172501));
#29758=CARTESIAN_POINT('Ctrl Pts',(-1.95664660002685,-6.1338053014481,8.50319674020009));
#29759=CARTESIAN_POINT('Ctrl Pts',(-1.89926159565089,-9.33896099596043,
4.68011416312611));
#29760=CARTESIAN_POINT('Ctrl Pts',(-1.86162611218989,-10.0616026543616,
1.50724548874808));
#29761=CARTESIAN_POINT('Ctrl Pts',(-1.84374014964383,-10.06270133709,-0.000151152320359421));
#29762=CARTESIAN_POINT('Origin',(-9.65625985035617,0.,0.));
#29763=CARTESIAN_POINT('',(-3.34374014964383,-10.0613110750442,-0.000128831358185422));
#29764=CARTESIAN_POINT('',(-3.28125985035617,-10.0619030430615,-0.000253284982714122));
#29765=CARTESIAN_POINT('',(-9.65625985035617,-10.06205,-4.69647557663214E-13));
#29766=CARTESIAN_POINT('Ctrl Pts',(-3.28125985035617,-10.0619030430615,
-0.000253284982714569));
#29767=CARTESIAN_POINT('Ctrl Pts',(-3.27613873944682,-10.0623258355878,
-0.431950106845118));
#29768=CARTESIAN_POINT('Ctrl Pts',(-3.25126810762252,-9.92988884013124,
-2.52822450542058));
#29769=CARTESIAN_POINT('Ctrl Pts',(-3.20664795488328,-8.50225392258195,
-6.13511212637845));
#29770=CARTESIAN_POINT('Ctrl Pts',(-3.14739939213844,-4.55450947899581,
-9.44374745389952));
#29771=CARTESIAN_POINT('Ctrl Pts',(-3.08815082939361,0.492492750162627,
-10.4730785091268));
#29772=CARTESIAN_POINT('Ctrl Pts',(-3.02890226664877,5.42062894282451,-8.97467015725421));
#29773=CARTESIAN_POINT('Ctrl Pts',(-2.96965370390394,9.04046429747557,-5.31017211146357));
#29774=CARTESIAN_POINT('Ctrl Pts',(-2.9104051411591,10.478330153541,-0.36403263684834));
#29775=CARTESIAN_POINT('Ctrl Pts',(-2.85115657841426,9.38718908708332,4.66996826655597));
#29776=CARTESIAN_POINT('Ctrl Pts',(-2.79190801566943,6.03039444449335,8.57684472350524));
#29777=CARTESIAN_POINT('Ctrl Pts',(-2.7326594529246,1.21812845559219,10.4136490066149));
#29778=CARTESIAN_POINT('Ctrl Pts',(-2.67341089017976,-3.88814003672063,
9.73705754435836));
#29779=CARTESIAN_POINT('Ctrl Pts',(-2.61416232743493,-8.05598294742662,
6.71036968564828));
#29780=CARTESIAN_POINT('Ctrl Pts',(-2.56677864749373,-9.83420068152227,
2.9945391385982));
#29781=CARTESIAN_POINT('Ctrl Pts',(-2.53914448846748,-10.0616829629283,
0.664906282705056));
#29782=CARTESIAN_POINT('Ctrl Pts',(-2.53125985035617,-10.0613414668576,
0.000144586642132558));
#29783=CARTESIAN_POINT('Ctrl Pts',(-3.34374014964383,-10.0613110750442,
-0.000128831358185907));
#29784=CARTESIAN_POINT('Ctrl Pts',(-3.33561461414857,-10.0616234356738,
-0.685206748448338));
#29785=CARTESIAN_POINT('Ctrl Pts',(-3.30773955773836,-9.82504498752015,
-3.03518808148316));
#29786=CARTESIAN_POINT('Ctrl Pts',(-3.26011498041321,-8.01520819574961,
-6.75902062856823));
#29787=CARTESIAN_POINT('Ctrl Pts',(-3.20086641766838,-3.82911697615253,
-9.76041932816225));
#29788=CARTESIAN_POINT('Ctrl Pts',(-3.14161785492354,1.28115426048353,-10.4060831266845));
#29789=CARTESIAN_POINT('Ctrl Pts',(-3.08236929217871,6.08221134313651,-8.54017724968541));
#29790=CARTESIAN_POINT('Ctrl Pts',(-3.02312072943387,9.41529076468844,-4.61304911040355));
#29791=CARTESIAN_POINT('Ctrl Pts',(-2.96387216668904,10.4759341041022,0.427465700532903));
#29792=CARTESIAN_POINT('Ctrl Pts',(-2.9046236039442,9.00814882168857,5.36480913779172));
#29793=CARTESIAN_POINT('Ctrl Pts',(-2.84537504119937,5.36619357179512,9.00732417694884));
#29794=CARTESIAN_POINT('Ctrl Pts',(-2.78612647845453,0.429075782469587,
10.4758682815087));
#29795=CARTESIAN_POINT('Ctrl Pts',(-2.7268779157097,-4.61160198332664,9.41599965091337));
#29796=CARTESIAN_POINT('Ctrl Pts',(-2.66762935296486,-8.5392423501426,6.08352384429894));
#29797=CARTESIAN_POINT('Ctrl Pts',(-2.62325009760957,-9.93742410704811,
2.48757824070357));
#29798=CARTESIAN_POINT('Ctrl Pts',(-2.59862036316923,-10.0623746461297,
0.411637313372905));
#29799=CARTESIAN_POINT('Ctrl Pts',(-2.59374014964383,-10.0619647730755,
0.000254798100391383));
#29800=CARTESIAN_POINT('Origin',(-9.65625985035617,0.,0.));
#29801=CARTESIAN_POINT('',(-4.09374014964383,-10.0627834482744,-0.000116052230568764));
#29802=CARTESIAN_POINT('',(-4.03125985035617,-10.0627446112277,0.000134087670397226));
#29803=CARTESIAN_POINT('',(-9.65625985035617,-10.06205,-4.69647557663214E-13));
#29804=CARTESIAN_POINT('Ctrl Pts',(-4.03125985035617,-10.0627446112277,
0.000134087670397437));
#29805=CARTESIAN_POINT('Ctrl Pts',(-4.01313299042616,-10.0617332034697,
-1.52754589633415));
#29806=CARTESIAN_POINT('Ctrl Pts',(-3.9752566095812,-9.32400657210876,-4.72060274017016));
#29807=CARTESIAN_POINT('Ctrl Pts',(-3.91763070782129,-6.08221135112264,
-8.54017726089867));
#29808=CARTESIAN_POINT('Ctrl Pts',(-3.85838214507646,-1.28115426216585,
-10.4060831403478));
#29809=CARTESIAN_POINT('Ctrl Pts',(-3.79913358233163,3.8291169811801,-9.76041934097784));
#29810=CARTESIAN_POINT('Ctrl Pts',(-3.73988501958678,8.01520820627361,-6.75902063744299));
#29811=CARTESIAN_POINT('Ctrl Pts',(-3.68063645684196,10.2667815509319,-2.12629234884133));
#29812=CARTESIAN_POINT('Ctrl Pts',(-3.62138789409711,10.0404064788223,3.01962916718597));
#29813=CARTESIAN_POINT('Ctrl Pts',(-3.56213933135229,7.39071995175672,7.43674533394825));
#29814=CARTESIAN_POINT('Ctrl Pts',(-3.50289076860744,2.95723947598601,10.0589590539462));
#29815=CARTESIAN_POINT('Ctrl Pts',(-3.44364220586262,-2.18998822827795,
10.2533835453132));
#29816=CARTESIAN_POINT('Ctrl Pts',(-3.38439364311777,-6.80864932809227,
7.97309330776734));
#29817=CARTESIAN_POINT('Ctrl Pts',(-3.3302661912823,-9.52682993830807,4.13187548496956));
#29818=CARTESIAN_POINT('Ctrl Pts',(-3.29588826036176,-10.0606953397857,
1.23288503599762));
#29819=CARTESIAN_POINT('Ctrl Pts',(-3.28125985035617,-10.0619030430615,
-0.000253284982714569));
#29820=CARTESIAN_POINT('Ctrl Pts',(-4.09374014964383,-10.0627834482744,
-0.00011605223056925));
#29821=CARTESIAN_POINT('Ctrl Pts',(-4.09235838604285,-10.0628518624021,
-0.11656583648092));
#29822=CARTESIAN_POINT('Ctrl Pts',(-4.07122710152693,-10.032574667649,-1.89739454732072));
#29823=CARTESIAN_POINT('Ctrl Pts',(-4.03034629609606,-9.04046428560539,
-5.31017210449113));
#29824=CARTESIAN_POINT('Ctrl Pts',(-3.97109773335123,-5.42062893570726,
-8.9746701454703));
#29825=CARTESIAN_POINT('Ctrl Pts',(-3.9118491706064,-0.492492749516077,
-10.4730784953755));
#29826=CARTESIAN_POINT('Ctrl Pts',(-3.85260060786156,4.5545094730156,-9.4437474414998));
#29827=CARTESIAN_POINT('Ctrl Pts',(-3.79335204511673,8.50225391141831,-6.13511211832306));
#29828=CARTESIAN_POINT('Ctrl Pts',(-3.73410348237189,10.3979291094031,-1.34573121924465));
#29829=CARTESIAN_POINT('Ctrl Pts',(-3.67485491962706,9.78400265213786,3.76844986454401));
#29830=CARTESIAN_POINT('Ctrl Pts',(-3.61560635688222,6.80864931915254,7.97309329729851));
#29831=CARTESIAN_POINT('Ctrl Pts',(-3.55635779413739,2.18998822540255,10.2533835318504));
#29832=CARTESIAN_POINT('Ctrl Pts',(-3.49710923139255,-2.95723947210302,
10.0589590407387));
#29833=CARTESIAN_POINT('Ctrl Pts',(-3.43786066864772,-7.39071994205252,
7.43674532418379));
#29834=CARTESIAN_POINT('Ctrl Pts',(-3.38673764139814,-9.67702006601549,
3.62540645957803));
#29835=CARTESIAN_POINT('Ctrl Pts',(-3.35536413506351,-10.0608642275218,
0.979909434950409));
#29836=CARTESIAN_POINT('Ctrl Pts',(-3.34374014964383,-10.0613110750442,
-0.000128831358185907));
#29837=CARTESIAN_POINT('Origin',(-9.65625985035617,0.,0.));
#29838=CARTESIAN_POINT('',(-4.84374014964383,-10.0618424730707,0.000250336541640639));
#29839=CARTESIAN_POINT('',(-4.78125985035617,-10.0612843796716,0.000112408078518301));
#29840=CARTESIAN_POINT('',(-9.65625985035617,-10.06205,-4.69647557663214E-13));
#29841=CARTESIAN_POINT('Ctrl Pts',(-4.78125985035617,-10.0612843796716,
0.000112408078517881));
#29842=CARTESIAN_POINT('Ctrl Pts',(-4.76987676232044,-10.0609038653183,
-0.959622679855897));
#29843=CARTESIAN_POINT('Ctrl Pts',(-4.73874415336977,-9.68812791873437,
-3.58477606207291));
#29844=CARTESIAN_POINT('Ctrl Pts',(-4.68786202350414,-7.43560933766978,
-7.3918628467291));
#29845=CARTESIAN_POINT('Ctrl Pts',(-4.62861346075931,-3.01808598246791,
-10.0408704587663));
#29846=CARTESIAN_POINT('Ctrl Pts',(-4.56936489801447,2.12787026524513,-10.2664546315455));
#29847=CARTESIAN_POINT('Ctrl Pts',(-4.51011633526964,6.76025244608102,-8.01416929148315));
#29848=CARTESIAN_POINT('Ctrl Pts',(-4.4508677725248,9.7610077375538,-3.82761681921153));
#29849=CARTESIAN_POINT('Ctrl Pts',(-4.39161920977998,10.4058861118699,1.28275359835361));
#29850=CARTESIAN_POINT('Ctrl Pts',(-4.33237064703513,8.53924236135476,6.08352385228661));
#29851=CARTESIAN_POINT('Ctrl Pts',(-4.2731220842903,4.61160198938182,9.41599966327665));
#29852=CARTESIAN_POINT('Ctrl Pts',(-4.21387352154547,-0.429075783032848,
10.4758682952637));
#29853=CARTESIAN_POINT('Ctrl Pts',(-4.15462495880063,-5.3661935788409,9.00732418877565));
#29854=CARTESIAN_POINT('Ctrl Pts',(-4.09537639605579,-9.00814883351634,
5.36480914483585));
#29855=CARTESIAN_POINT('Ctrl Pts',(-4.05425469324098,-10.02687110225,1.93802610770741));
#29856=CARTESIAN_POINT('Ctrl Pts',(-4.0328825113411,-10.0628351493527,0.136887321108126));
#29857=CARTESIAN_POINT('Ctrl Pts',(-4.03125985035617,-10.0627446112277,
0.000134087670397437));
#29858=CARTESIAN_POINT('Ctrl Pts',(-4.84374014964383,-10.0618424730707,
0.00025033654164057));
#29859=CARTESIAN_POINT('Ctrl Pts',(-4.8293526370222,-10.0606807693026,-1.2126019193507));
#29860=CARTESIAN_POINT('Ctrl Pts',(-4.79521560348561,-9.53967754434127,
-4.09128924672136));
#29861=CARTESIAN_POINT('Ctrl Pts',(-4.74132904903408,-6.85679662469408,
-7.93172505361893));
#29862=CARTESIAN_POINT('Ctrl Pts',(-4.68208048628925,-2.25202591260958,
-10.2399365997821));
#29863=CARTESIAN_POINT('Ctrl Pts',(-4.62283192354441,2.89628456575783,-10.0766789168245));
#29864=CARTESIAN_POINT('Ctrl Pts',(-4.56358336079958,7.34555964353492,-7.48135521158391));
#29865=CARTESIAN_POINT('Ctrl Pts',(-4.50433479805474,10.0219404799498,-3.08036220191168));
#29866=CARTESIAN_POINT('Ctrl Pts',(-4.44508623530991,10.2794667393936,2.0640944339644));
#29867=CARTESIAN_POINT('Ctrl Pts',(-4.38583767256508,8.0559829368491,6.71036967683738));
#29868=CARTESIAN_POINT('Ctrl Pts',(-4.32658910982024,3.88814003161556,9.73705753157345));
#29869=CARTESIAN_POINT('Ctrl Pts',(-4.2673405470754,-1.21812845399267,10.4136489929417));
#29870=CARTESIAN_POINT('Ctrl Pts',(-4.20809198433057,-6.03039443657531,
8.57684471224378));
#29871=CARTESIAN_POINT('Ctrl Pts',(-4.15022518518671,-9.30890368803934,
4.76108236386482));
#29872=CARTESIAN_POINT('Ctrl Pts',(-4.1121079069578,-10.061874020574,1.54784871892385));
#29873=CARTESIAN_POINT('Ctrl Pts',(-4.09374014964383,-10.0627834482744,
-0.00011605223056925));
#29874=CARTESIAN_POINT('Origin',(-9.65625985035617,0.,0.));
#29875=CARTESIAN_POINT('',(-5.59374014964383,-10.061375386696,-0.000159589291578444));
#29876=CARTESIAN_POINT('',(-5.53125985035618,-10.0620274206975,-0.000254850986975038));
#29877=CARTESIAN_POINT('',(-9.65625985035617,-10.06205,-4.69647557663214E-13));
#29878=CARTESIAN_POINT('Ctrl Pts',(-5.53125985035617,-10.0620274206975,
-0.000254850986975523));
#29879=CARTESIAN_POINT('Ctrl Pts',(-5.52662053421473,-10.0624218030828,
-0.391323674499798));
#29880=CARTESIAN_POINT('Ctrl Pts',(-5.50223169715834,-9.94483149077408,
-2.44693269826794));
#29881=CARTESIAN_POINT('Ctrl Pts',(-5.458093339187,-8.57591778746981,-6.03171258183405));
#29882=CARTESIAN_POINT('Ctrl Pts',(-5.39884477644216,-4.6685254578629,-9.38790672176614));
#29883=CARTESIAN_POINT('Ctrl Pts',(-5.33959621369733,0.365643087792113,
-10.4782740801931));
#29884=CARTESIAN_POINT('Ctrl Pts',(-5.2803476509525,5.31156151280302,-9.03964804973101));
#29885=CARTESIAN_POINT('Ctrl Pts',(-5.22109908820765,8.975503168763,-5.41924952690144));
#29886=CARTESIAN_POINT('Ctrl Pts',(-5.16185052546283,10.4731540785531,-0.490883096248158));
#29887=CARTESIAN_POINT('Ctrl Pts',(-5.10260196271799,9.44304734211565,4.55596087141438));
#29888=CARTESIAN_POINT('Ctrl Pts',(-5.04335339997316,6.13380530950194,8.50319675136485));
#29889=CARTESIAN_POINT('Ctrl Pts',(-4.98410483722832,1.34413310702038,10.3981358309029));
#29890=CARTESIAN_POINT('Ctrl Pts',(-4.92485627448348,-3.76995356633927,
9.78342336173498));
#29891=CARTESIAN_POINT('Ctrl Pts',(-4.86560771173865,-7.97413966134769,
6.80742383201003));
#29892=CARTESIAN_POINT('Ctrl Pts',(-4.81774223702955,-9.81575725621947,
3.07583662613618));
#29893=CARTESIAN_POINT('Ctrl Pts',(-4.78962628323539,-10.0615640531474,
0.705506161498075));
#29894=CARTESIAN_POINT('Ctrl Pts',(-4.78125985035617,-10.0612843796716,
0.000112408078517881));
#29895=CARTESIAN_POINT('Ctrl Pts',(-5.59374014964383,-10.061375386696,-0.000159589291578652));
#29896=CARTESIAN_POINT('Ctrl Pts',(-5.58609640891648,-10.0617424196366,
-0.64460476064184));
#29897=CARTESIAN_POINT('Ctrl Pts',(-5.55870314727419,-9.84322461794499,
-2.95388988874244));
#29898=CARTESIAN_POINT('Ctrl Pts',(-5.51156036471693,-8.09646237954581,
-6.66147275121817));
#29899=CARTESIAN_POINT('Ctrl Pts',(-5.4523118019721,-3.94702056424182,-9.71333881546786));
#29900=CARTESIAN_POINT('Ctrl Pts',(-5.39306323922727,1.15505799604341,-10.420833138689));
#29901=CARTESIAN_POINT('Ctrl Pts',(-5.33381467648243,5.97835648115395,-8.61319778380056));
#29902=CARTESIAN_POINT('Ctrl Pts',(-5.27456611373759,9.35874329001436,-4.72671622907851));
#29903=CARTESIAN_POINT('Ctrl Pts',(-5.21531755099276,10.480342084015,0.300586228304444));
#29904=CARTESIAN_POINT('Ctrl Pts',(-5.15606898824793,9.07244836417983,5.25534042264758));
#29905=CARTESIAN_POINT('Ctrl Pts',(-5.09682042550309,5.47486560219418,8.9416871403854));
#29906=CARTESIAN_POINT('Ctrl Pts',(-5.03757186275826,0.555891663852748,
10.4699048102971));
#29907=CARTESIAN_POINT('Ctrl Pts',(-4.97832330001342,-4.49725001357077,
9.47114906408194));
#29908=CARTESIAN_POINT('Ctrl Pts',(-4.91907473726859,-8.464953815877,6.18647550497794));
#29909=CARTESIAN_POINT('Ctrl Pts',(-4.87421368714539,-9.92222535333499,
2.5688714186231));
#29910=CARTESIAN_POINT('Ctrl Pts',(-4.84910215793714,-10.0622754224904,
0.452262023737051));
#29911=CARTESIAN_POINT('Ctrl Pts',(-4.84374014964383,-10.0618424730707,
0.00025033654164057));
#29912=CARTESIAN_POINT('Origin',(-9.65625985035617,0.,0.));
#29913=CARTESIAN_POINT('',(-6.34374014964383,-10.0628459703277,-7.75181276524428E-5));
#29914=CARTESIAN_POINT('',(-6.28125985035617,-10.0626541504143,0.000167148211893109));
#29915=CARTESIAN_POINT('',(-9.65625985035617,-10.06205,-4.69647557663214E-13));
#29916=CARTESIAN_POINT('Ctrl Pts',(-6.28125985035617,-10.0626541504143,
0.000167148211892981));
#29917=CARTESIAN_POINT('Ctrl Pts',(-6.26361478519406,-10.0614821172421,
-1.48694732055795));
#29918=CARTESIAN_POINT('Ctrl Pts',(-6.22622019911701,-9.35376745039498,
-4.63961696798018));
#29919=CARTESIAN_POINT('Ctrl Pts',(-6.16907609212502,-6.18517442841409,
-8.46590455045353));
#29920=CARTESIAN_POINT('Ctrl Pts',(-6.10982752938018,-1.40706268161673,
-10.3898073695953));
#29921=CARTESIAN_POINT('Ctrl Pts',(-6.05057896663535,3.71065196087965,-9.80606876339935));
#29922=CARTESIAN_POINT('Ctrl Pts',(-5.99133040389051,7.93277881804871,-6.85557749509213));
#29923=CARTESIAN_POINT('Ctrl Pts',(-5.93208184114569,10.2402826148908,-2.25045207335339));
#29924=CARTESIAN_POINT('Ctrl Pts',(-5.87283327840083,10.0762336698203,2.89783325926043));
#29925=CARTESIAN_POINT('Ctrl Pts',(-5.81358471565602,7.4802261654632,7.34670940495238));
#29926=CARTESIAN_POINT('Ctrl Pts',(-5.75433615291117,3.07882185862981,10.0224138075675));
#29927=CARTESIAN_POINT('Ctrl Pts',(-5.69508759016634,-2.06567430345103,
10.2791493927931));
#29928=CARTESIAN_POINT('Ctrl Pts',(-5.63583902742151,-6.7116077616892,8.05495150950825));
#29929=CARTESIAN_POINT('Ctrl Pts',(-5.58122978081811,-9.50070766399809,
4.21303279626446));
#29930=CARTESIAN_POINT('Ctrl Pts',(-5.54637005512967,-10.0607429213405,
1.27345226955577));
#29931=CARTESIAN_POINT('Ctrl Pts',(-5.53125985035617,-10.0620274206975,
-0.000254850986975523));
#29932=CARTESIAN_POINT('Ctrl Pts',(-6.34374014964383,-10.0628459703277,
-7.75181276522433E-5));
#29933=CARTESIAN_POINT('Ctrl Pts',(-6.34284018081076,-10.0628773940367,
-0.0759221005433881));
#29934=CARTESIAN_POINT('Ctrl Pts',(-6.32219069106275,-10.0436093238266,
-1.81613516389724));
#29935=CARTESIAN_POINT('Ctrl Pts',(-6.28179168039979,-9.10409988500852,
-5.20031610215367));
#29936=CARTESIAN_POINT('Ctrl Pts',(-6.22254311765495,-5.52890158316907,
-8.90837637071521));
#29937=CARTESIAN_POINT('Ctrl Pts',(-6.16329455491012,-0.61927020154201,
-10.4663473426058));
#29938=CARTESIAN_POINT('Ctrl Pts',(-6.10404599216529,4.43982570388255,-9.49820351423256));
#29939=CARTESIAN_POINT('Ctrl Pts',(-6.04479742942044,8.42734343078316,-6.23761212149772));
#29940=CARTESIAN_POINT('Ctrl Pts',(-5.98554886667563,10.3808720045808,-1.47153617119417));
#29941=CARTESIAN_POINT('Ctrl Pts',(-5.92630030393077,9.82891575620613,3.64970373263731));
#29942=CARTESIAN_POINT('Ctrl Pts',(-5.86705174118595,6.90469258895211,7.89006606630713));
#29943=CARTESIAN_POINT('Ctrl Pts',(-5.80780317844112,2.31398105003217,10.2261143147686));
#29944=CARTESIAN_POINT('Ctrl Pts',(-5.74855461569627,-2.83522349381956,
10.094029424304));
#29945=CARTESIAN_POINT('Ctrl Pts',(-5.68930605295145,-7.3001300877402,7.5256908640133));
#29946=CARTESIAN_POINT('Ctrl Pts',(-5.63770123093395,-9.65439224755071,
3.70665976616409));
#29947=CARTESIAN_POINT('Ctrl Pts',(-5.60584592983142,-10.0607940979973,
1.020480940731));
#29948=CARTESIAN_POINT('Ctrl Pts',(-5.59374014964383,-10.061375386696,-0.000159589291578652));
#29949=CARTESIAN_POINT('Origin',(-9.65625985035617,0.,0.));
#29950=CARTESIAN_POINT('',(-7.09374014964383,-10.0617260250247,0.000240284390234935));
#29951=CARTESIAN_POINT('',(-7.03125985035617,-10.0612423609455,7.79087254440521E-5));
#29952=CARTESIAN_POINT('',(-9.65625985035617,-10.06205,-4.69647557663214E-13));
#29953=CARTESIAN_POINT('Ctrl Pts',(-7.03125985035617,-10.0612423609455,
7.79087254439148E-5));
#29954=CARTESIAN_POINT('Ctrl Pts',(-7.02035855708835,-10.0609911152643,
-0.919046910462609));
#29955=CARTESIAN_POINT('Ctrl Pts',(-6.98970774290558,-9.70993335321315,
-3.50350861223781));
#29956=CARTESIAN_POINT('Ctrl Pts',(-6.93930740780787,-7.52456879985629,
-7.30128666317293));
#29957=CARTESIAN_POINT('Ctrl Pts',(-6.88005884506304,-3.13944487805482,
-10.0035897771931));
#29958=CARTESIAN_POINT('Ctrl Pts',(-6.8208102823182,2.0034026226881,-10.2914673635639));
#29959=CARTESIAN_POINT('Ctrl Pts',(-6.76156171957337,6.6627170580516,-8.09543846701894));
#29960=CARTESIAN_POINT('Ctrl Pts',(-6.70231315682853,9.71394534640064,-3.94552764200815));
#29961=CARTESIAN_POINT('Ctrl Pts',(-6.6430645940837,10.4206555039509,1.1566596022022));
#29962=CARTESIAN_POINT('Ctrl Pts',(-6.58381603133886,8.61227885655681,5.97968021421488));
#29963=CARTESIAN_POINT('Ctrl Pts',(-6.52456746859403,4.72527779786631,9.35946965913116));
#29964=CARTESIAN_POINT('Ctrl Pts',(-6.46531890584919,-0.302196989616849,
10.480295775732));
#29965=CARTESIAN_POINT('Ctrl Pts',(-6.40607034310435,-5.25673474729183,
9.07164055526217));
#29966=CARTESIAN_POINT('Ctrl Pts',(-6.34682178035952,-8.94252849986846,
5.4734912621059));
#29967=CARTESIAN_POINT('Ctrl Pts',(-6.30521828277679,-10.015090324262,2.01929287385976));
#29968=CARTESIAN_POINT('Ctrl Pts',(-6.28336430610901,-10.0627939340835,
0.177529292821701));
#29969=CARTESIAN_POINT('Ctrl Pts',(-6.28125985035617,-10.0626541504143,
0.000167148211892981));
#29970=CARTESIAN_POINT('Ctrl Pts',(-7.09374014964383,-10.0617260250247,
0.00024028439023438));
#29971=CARTESIAN_POINT('Ctrl Pts',(-7.0798344317901,-10.0606687753925,-1.17203615203383));
#29972=CARTESIAN_POINT('Ctrl Pts',(-7.04617919302143,-9.56494781223263,
-4.01010281132586));
#29973=CARTESIAN_POINT('Ctrl Pts',(-6.9927744333378,-6.95233545178506,-7.84811784659899));
#29974=CARTESIAN_POINT('Ctrl Pts',(-6.93352587059297,-2.37585136897494,
-10.2119171916642));
#29975=CARTESIAN_POINT('Ctrl Pts',(-6.87427730784814,2.77405849573116,-10.1110099229398));
#29976=CARTESIAN_POINT('Ctrl Pts',(-6.8150287451033,7.25443293930229,-7.56975065851036));
#29977=CARTESIAN_POINT('Ctrl Pts',(-6.75578018235847,9.98390711286757,-3.20148731676458));
#29978=CARTESIAN_POINT('Ctrl Pts',(-6.69653161961363,10.3037062860758,1.93947390886785));
#29979=CARTESIAN_POINT('Ctrl Pts',(-6.63728305686881,8.13664504012033,6.61233164437115));
#29980=CARTESIAN_POINT('Ctrl Pts',(-6.57803449412396,4.00575641567419,9.68926404911563));
#29981=CARTESIAN_POINT('Ctrl Pts',(-6.51878593137913,-1.09194519850991,
10.4276353006677));
#29982=CARTESIAN_POINT('Ctrl Pts',(-6.45953736863429,-5.92609938437677,
8.64923513176283));
#29983=CARTESIAN_POINT('Ctrl Pts',(-6.40118877472253,-9.27825086183916,
4.84201353009798));
#29984=CARTESIAN_POINT('Ctrl Pts',(-6.3625897017257,-10.0621878110463,1.58846238885859));
#29985=CARTESIAN_POINT('Ctrl Pts',(-6.34374014964383,-10.0628459703277,
-7.75181276522433E-5));
#29986=CARTESIAN_POINT('Origin',(-9.65625985035617,0.,0.));
#29987=CARTESIAN_POINT('',(-7.84374014964383,-10.0614619079128,-0.000218150500570502));
#29988=CARTESIAN_POINT('',(-7.78125985035617,-10.0621541710632,-0.000250329009834688));
#29989=CARTESIAN_POINT('',(-9.65625985035617,-10.06205,-4.69647557663214E-13));
#29990=CARTESIAN_POINT('',(-8.,-2.60344811511687,9.71940883564398));
#29991=CARTESIAN_POINT('Ctrl Pts',(-8.,-2.60344811511687,9.71940883564398));
#29992=CARTESIAN_POINT('Ctrl Pts',(-7.98025047908506,-4.2115554043733,9.28866001522532));
#29993=CARTESIAN_POINT('Ctrl Pts',(-7.94075143725516,-7.20829614504029,
7.61418486945486));
#29994=CARTESIAN_POINT('Ctrl Pts',(-7.88866482046978,-9.63126793254245,
3.78770677709999));
#29995=CARTESIAN_POINT('Ctrl Pts',(-7.85632772459933,-10.0607601076051,
1.06096981025071));
#29996=CARTESIAN_POINT('Ctrl Pts',(-7.84374014964383,-10.0614619079128,
-0.000218150500570363));
#29997=CARTESIAN_POINT('',(-8.,2.6037558201701,9.72001092048762));
#29998=CARTESIAN_POINT('Origin',(-8.,0.,0.));
#29999=CARTESIAN_POINT('Ctrl Pts',(-8.,2.6037558201701,9.72001092048762));
#30000=CARTESIAN_POINT('Ctrl Pts',(-7.98217765815669,1.15257245541084,10.107573988037));
#30001=CARTESIAN_POINT('Ctrl Pts',(-7.94460579539843,-2.09302813938078,
10.2328568518709));
#30002=CARTESIAN_POINT('Ctrl Pts',(-7.88728441172523,-6.61358902169624,
8.13565037958078));
#30003=CARTESIAN_POINT('Ctrl Pts',(-7.83219337035393,-9.47401039595774,
4.29415937030418));
#30004=CARTESIAN_POINT('Ctrl Pts',(-7.79685184989758,-10.0608163520868,
1.3140197112117));
#30005=CARTESIAN_POINT('Ctrl Pts',(-7.78125985035617,-10.0621541710632,
-0.000250329009834835));
#30006=CARTESIAN_POINT('Origin',(-9.65625985035617,0.,0.));
#30007=CARTESIAN_POINT('Ctrl Pts',(-7.78125985035617,-10.0621541710632,
-0.000250329009834835));
#30008=CARTESIAN_POINT('Ctrl Pts',(-7.77710232898263,-10.062510893174,-0.350693244834193));
#30009=CARTESIAN_POINT('Ctrl Pts',(-7.75319528669415,-9.95926473270352,
-2.36564048511104));
#30010=CARTESIAN_POINT('Ctrl Pts',(-7.70953872349072,-8.64832327843871,
-5.92743166991522));
#30011=CARTESIAN_POINT('Ctrl Pts',(-7.65029016074589,-4.78185742483636,
-9.33068795739798));
#30012=CARTESIAN_POINT('Ctrl Pts',(-7.59104159800105,0.238740070891225,
-10.4819341157898));
#30013=CARTESIAN_POINT('Ctrl Pts',(-7.53179303525622,5.20171515908679,-9.10330011423497));
#30014=CARTESIAN_POINT('Ctrl Pts',(-7.47254447251139,8.90922610438627,-5.52753257885261));
#30015=CARTESIAN_POINT('Ctrl Pts',(-7.41329590976654,10.4664423751253,-0.617661469275298));
#30016=CARTESIAN_POINT('Ctrl Pts',(-7.35404734702172,9.49752105893024,4.4412854149463));
#30017=CARTESIAN_POINT('Ctrl Pts',(-7.29479878427687,6.23631681532395,8.42830205522834));
#30018=CARTESIAN_POINT('Ctrl Pts',(-7.23555022153205,1.46994068417205,10.38109804613));
#30019=CARTESIAN_POINT('Ctrl Pts',(-7.17630165878721,-3.65121434111183,
9.82835472395443));
#30020=CARTESIAN_POINT('Ctrl Pts',(-7.11705309604238,-7.89112719116351,
6.90347985740062));
#30021=CARTESIAN_POINT('Ctrl Pts',(-7.06870582656536,-9.79678423589676,
3.15713204118938));
#30022=CARTESIAN_POINT('Ctrl Pts',(-7.0401080780033,-10.06144628895,0.746101837858744));
#30023=CARTESIAN_POINT('Ctrl Pts',(-7.03125985035617,-10.0612423609455,
7.79087254439148E-5));
#30024=CARTESIAN_POINT('Ctrl Pts',(-7.84374014964383,-10.0614619079128,
-0.000218150500570363));
#30025=CARTESIAN_POINT('Ctrl Pts',(-7.83657820368438,-10.0618612108679,
-0.60400171124062));
#30026=CARTESIAN_POINT('Ctrl Pts',(-7.80966673680999,-9.86084825550603,
-2.87248335114659));
#30027=CARTESIAN_POINT('Ctrl Pts',(-7.76300574902067,-8.17655263057037,
-6.56303005806257));
#30028=CARTESIAN_POINT('Ctrl Pts',(-7.70375718627582,-4.06433342707358,
-9.66479172255802));
#30029=CARTESIAN_POINT('Ctrl Pts',(-7.644508623531,1.02878615653537,-10.4340771844272));
#30030=CARTESIAN_POINT('Ctrl Pts',(-7.58526006078616,5.87362828262073,-8.68494406353048));
#30031=CARTESIAN_POINT('Ctrl Pts',(-7.52601149804132,9.30082195115954,-4.83969619824767));
#30032=CARTESIAN_POINT('Ctrl Pts',(-7.46676293529649,10.483214281353,0.173665734501785));
#30033=CARTESIAN_POINT('Ctrl Pts',(-7.40751437255165,9.13541724029078,5.1450995797055));
#30034=CARTESIAN_POINT('Ctrl Pts',(-7.34826580980682,5.58273512973762,8.87473987601911));
#30035=CARTESIAN_POINT('Ctrl Pts',(-7.28901724706198,0.682625919309218,
10.4624057987323));
#30036=CARTESIAN_POINT('Ctrl Pts',(-7.22976868431715,-4.38223858668436,
9.52491001985317));
#30037=CARTESIAN_POINT('Ctrl Pts',(-7.17052012157231,-8.38942416699272,
6.28851997968158));
#30038=CARTESIAN_POINT('Ctrl Pts',(-7.1251772766812,-9.90651266144331,2.65016697566111));
#30039=CARTESIAN_POINT('Ctrl Pts',(-7.09958395270504,-10.0621703284905,
0.49288314539355));
#30040=CARTESIAN_POINT('Ctrl Pts',(-7.09374014964383,-10.0617260250247,
0.00024028439023438));
#30041=CARTESIAN_POINT('Ctrl Pts',(-8.,7.21801009705396,-6.39216838336781));
#30042=CARTESIAN_POINT('Ctrl Pts',(-7.98025047908506,8.27561480792393,-5.19792551867511));
#30043=CARTESIAN_POINT('Ctrl Pts',(-7.94075143725517,9.78570906708942,-2.27567127227239));
#30044=CARTESIAN_POINT('Ctrl Pts',(-7.88150287451033,9.68796046702948,2.65991246200497));
#30045=CARTESIAN_POINT('Ctrl Pts',(-7.8222543117655,7.25238499100985,6.95222960735294));
#30046=CARTESIAN_POINT('Ctrl Pts',(-7.76300574902066,3.06619992068337,9.56722174110869));
#30047=CARTESIAN_POINT('Ctrl Pts',(-7.70375718627582,-1.85992661552226,
9.87278141350118));
#30048=CARTESIAN_POINT('Ctrl Pts',(-7.64450862353099,-6.33720258119721,
7.79565594657622));
#30049=CARTESIAN_POINT('Ctrl Pts',(-7.58526006078615,-9.28492944394566,
3.83691534180259));
#30050=CARTESIAN_POINT('Ctrl Pts',(-7.52601149804132,-9.99169809387859,
-1.04784215725893));
#30051=CARTESIAN_POINT('Ctrl Pts',(-7.46676293529649,-8.28690389187399,
-5.67972021775593));
#30052=CARTESIAN_POINT('Ctrl Pts',(-7.40751437255165,-4.58202030942313,
-8.94075208090305));
#30053=CARTESIAN_POINT('Ctrl Pts',(-7.34826580980682,0.228762958890216,
-10.0438868693848));
#30054=CARTESIAN_POINT('Ctrl Pts',(-7.28901724706198,4.98433189977125,-8.72286693232514));
#30055=CARTESIAN_POINT('Ctrl Pts',(-7.22976868431715,8.53690340902155,-5.29653318514979));
#30056=CARTESIAN_POINT('Ctrl Pts',(-7.17052012157231,10.0290425392331,-0.591848971043799));
#30057=CARTESIAN_POINT('Ctrl Pts',(-7.11127155882747,9.10061311221161,4.25568103840426));
#30058=CARTESIAN_POINT('Ctrl Pts',(-7.05202299608264,5.97569684018532,8.07607750712695));
#30059=CARTESIAN_POINT('Ctrl Pts',(-6.99277443333781,1.40851085052043,9.94726480852957));
#30060=CARTESIAN_POINT('Ctrl Pts',(-6.93352587059297,-3.49862757892743,
9.4176210105041));
#30061=CARTESIAN_POINT('Ctrl Pts',(-6.87427730784813,-7.56135155062463,
6.61497867920762));
#30062=CARTESIAN_POINT('Ctrl Pts',(-6.8150287451033,-9.79909863393696,2.21577215777723));
#30063=CARTESIAN_POINT('Ctrl Pts',(-6.75578018235847,-9.67177533431446,
-2.71822408062585));
#30064=CARTESIAN_POINT('Ctrl Pts',(-6.69653161961363,-7.21011188696681,
-6.99616086456685));
#30065=CARTESIAN_POINT('Ctrl Pts',(-6.6372830568688,-3.00824531422618,-9.58553287017026));
#30066=CARTESIAN_POINT('Ctrl Pts',(-6.57803449412396,1.91967904719004,-9.8613798539234));
#30067=CARTESIAN_POINT('Ctrl Pts',(-6.51878593137913,6.38427752307505,-7.75712451753733));
#30068=CARTESIAN_POINT('Ctrl Pts',(-6.45953736863429,9.30799287964075,-3.78064132426331));
#30069=CARTESIAN_POINT('Ctrl Pts',(-6.40028880588946,9.98516913294189,1.10832200074663));
#30070=CARTESIAN_POINT('Ctrl Pts',(-6.34104024314462,8.2523657912091,5.72978525940176));
#30071=CARTESIAN_POINT('Ctrl Pts',(-6.28179168039979,4.52780518403485,8.96833097549665));
#30072=CARTESIAN_POINT('Ctrl Pts',(-6.22254311765496,-0.289567969274681,
10.0423169966864));
#30073=CARTESIAN_POINT('Ctrl Pts',(-6.16329455491011,-5.03705218148902,
8.69253044812817));
#30074=CARTESIAN_POINT('Ctrl Pts',(-6.10404599216529,-8.56881407445866,
5.24475029225229));
#30075=CARTESIAN_POINT('Ctrl Pts',(-6.04479742942045,-10.0324420382062,
0.531118650339597));
#30076=CARTESIAN_POINT('Ctrl Pts',(-5.98554886667561,-9.07468081182084,
-4.31070161740279));
#30077=CARTESIAN_POINT('Ctrl Pts',(-5.92630030393079,-5.92669172885007,
-8.11210856817701));
#30078=CARTESIAN_POINT('Ctrl Pts',(-5.86705174118593,-1.34826056300076,
-9.95561016336843));
#30079=CARTESIAN_POINT('Ctrl Pts',(-5.80780317844112,3.55558125962594,-9.39626639559069));
#30080=CARTESIAN_POINT('Ctrl Pts',(-5.74855461569627,7.60126252733364,-6.56907818961398));
#30081=CARTESIAN_POINT('Ctrl Pts',(-5.68930605295145,9.81233415115218,-2.15640413115026));
#30082=CARTESIAN_POINT('Ctrl Pts',(-5.6300574902066,9.65514092448912,2.77673081139753));
#30083=CARTESIAN_POINT('Ctrl Pts',(-5.57080892746178,7.16762236180716,7.03968535868123));
#30084=CARTESIAN_POINT('Ctrl Pts',(-5.51156036471693,2.95015577253862,9.60357023134971));
#30085=CARTESIAN_POINT('Ctrl Pts',(-5.45231180197211,-1.97934835152263,
9.84957665963537));
#30086=CARTESIAN_POINT('Ctrl Pts',(-5.39306323922727,-6.43112505053289,
7.71832953786746));
#30087=CARTESIAN_POINT('Ctrl Pts',(-5.33381467648243,-9.33071170264792,
3.72421795720638));
#30088=CARTESIAN_POINT('Ctrl Pts',(-5.27456611373759,-9.97827592921563,
-1.16875564218737));
#30089=CARTESIAN_POINT('Ctrl Pts',(-5.21531755099277,-8.21752427624387,
-5.77964315853947));
#30090=CARTESIAN_POINT('Ctrl Pts',(-5.15606898824792,-4.47342456340985,
-8.99557963369734));
#30091=CARTESIAN_POINT('Ctrl Pts',(-5.0968204255031,0.350362611307043,-10.0403797891966));
#30092=CARTESIAN_POINT('Ctrl Pts',(-5.03757186275825,5.08958769870612,-8.66187493143883));
#30093=CARTESIAN_POINT('Ctrl Pts',(-4.97832330001343,8.60041070922793,-5.19277535652244));
#30094=CARTESIAN_POINT('Ctrl Pts',(-4.91907473726859,10.0354737559517,-0.470368753547383));
#30095=CARTESIAN_POINT('Ctrl Pts',(-4.85982617452376,9.0484158895429,4.36556412856081));
#30096=CARTESIAN_POINT('Ctrl Pts',(-4.80057761177892,5.87746936079909,8.14784230232624));
#30097=CARTESIAN_POINT('Ctrl Pts',(-4.74132904903409,1.28796085867118,9.96359057254162));
#30098=CARTESIAN_POINT('Ctrl Pts',(-4.68208048628925,-3.61240461014787,
9.37456736085946));
#30099=CARTESIAN_POINT('Ctrl Pts',(-4.62283192354442,-7.64089487250279,
6.52293690127919));
#30100=CARTESIAN_POINT('Ctrl Pts',(-4.56358336079958,-9.8252099901855,2.0969570619038));
#30101=CARTESIAN_POINT('Ctrl Pts',(-4.50433479805475,-9.63815259752371,
-2.83513575998683));
#30102=CARTESIAN_POINT('Ctrl Pts',(-4.4450862353099,-7.12487010197824,-7.08295180702551));
#30103=CARTESIAN_POINT('Ctrl Pts',(-4.38583767256508,-2.89195809047495,
-9.62125556638245));
#30104=CARTESIAN_POINT('Ctrl Pts',(-4.32658910982023,2.03894510123426,-9.83741242120418));
#30105=CARTESIAN_POINT('Ctrl Pts',(-4.26734054707541,6.47773684005869,-7.67925163682345));
#30106=CARTESIAN_POINT('Ctrl Pts',(-4.20809198433056,9.35308850105216,-3.66765807596552));
#30107=CARTESIAN_POINT('Ctrl Pts',(-4.14884342158574,9.97101696392875,1.22914644194833));
#30108=CARTESIAN_POINT('Ctrl Pts',(-4.08959485884089,8.18238154144732,5.82928920031346));
#30109=CARTESIAN_POINT('Ctrl Pts',(-4.03034629609607,4.41887996588413,9.02249855183238));
#30110=CARTESIAN_POINT('Ctrl Pts',(-3.97109773335123,-0.411144410522746,
10.0380745436764));
#30111=CARTESIAN_POINT('Ctrl Pts',(-3.9118491706064,-5.14193665307501,8.63090190689669));
#30112=CARTESIAN_POINT('Ctrl Pts',(-3.85260060786156,-8.63169208916567,
5.14061007552062));
#30113=CARTESIAN_POINT('Ctrl Pts',(-3.79335204511673,-10.0381376154984,
0.409601615017363));
#30114=CARTESIAN_POINT('Ctrl Pts',(-3.73410348237189,-9.02181929045025,
-4.42026661652537));
#30115=CARTESIAN_POINT('Ctrl Pts',(-3.67485491962706,-5.82803154947716,
-8.18327737089536));
#30116=CARTESIAN_POINT('Ctrl Pts',(-3.61560635688222,-1.22761394312144,
-9.97120575845082));
#30117=CARTESIAN_POINT('Ctrl Pts',(-3.55635779413739,3.66909554513215,-9.35252469397438));
#30118=CARTESIAN_POINT('Ctrl Pts',(-3.49710923139255,7.68024713464924,-6.47655650955208));
#30119=CARTESIAN_POINT('Ctrl Pts',(-3.43786066864772,9.83772567840422,-2.0374331270438));
#30120=CARTESIAN_POINT('Ctrl Pts',(-3.37861210590288,9.6208109764798,2.89343678444073));
#30121=CARTESIAN_POINT('Ctrl Pts',(-3.31936354315805,7.08185667442123,7.12595862418978));
#30122=CARTESIAN_POINT('Ctrl Pts',(-3.26011498041321,2.83365440140854,9.63858822671076));
#30123=CARTESIAN_POINT('Ctrl Pts',(-3.20086641766838,-2.09846711180656,
9.82488758466862));
#30124=CARTESIAN_POINT('Ctrl Pts',(-3.14161785492354,-6.52411118303607,
7.63989224675928));
#30125=CARTESIAN_POINT('Ctrl Pts',(-3.08236929217871,-9.37512245462701,
3.61096375382772));
#30126=CARTESIAN_POINT('Ctrl Pts',(-3.02312072943387,-9.96339250315773,
-1.28949218637783));
#30127=CARTESIAN_POINT('Ctrl Pts',(-2.96387216668905,-8.14693887500758,
-5.87872156489823));
#30128=CARTESIAN_POINT('Ctrl Pts',(-2.9046236039442,-4.3641733908311,-9.04908674317308));
#30129=CARTESIAN_POINT('Ctrl Pts',(-2.84537504119937,0.471911138916074,
-10.0354013446237));
#30130=CARTESIAN_POINT('Ctrl Pts',(-2.78612647845453,5.19409712570397,-8.59961250984385));
#30131=CARTESIAN_POINT('Ctrl Pts',(-2.7268779157097,8.66265706762792,-5.08825636140564));
#30132=CARTESIAN_POINT('Ctrl Pts',(-2.66762935296487,10.0404335192006,-0.348819462217449));
#30133=CARTESIAN_POINT('Ctrl Pts',(-2.60838079022003,8.99489198946221,4.47480707613385));
#30134=CARTESIAN_POINT('Ctrl Pts',(-2.54913222747519,5.77838010706614,8.21841247498393));
#30135=CARTESIAN_POINT('Ctrl Pts',(-2.48988366473036,1.16722202841516,9.97845544195549));
#30136=CARTESIAN_POINT('Ctrl Pts',(-2.43063510198552,-3.72565198652797,
9.33013920292668));
#30137=CARTESIAN_POINT('Ctrl Pts',(-2.37138653924069,-7.71931787128481,
6.42993871454248));
#30138=CARTESIAN_POINT('Ctrl Pts',(-2.31213797649585,-9.8498807570359,1.97783450846704));
#30139=CARTESIAN_POINT('Ctrl Pts',(-2.25288941375102,-9.60311669702822,
-2.95163174768923));
#30140=CARTESIAN_POINT('Ctrl Pts',(-2.19364085100618,-7.03858365582718,
-7.16870423372533));
#30141=CARTESIAN_POINT('Ctrl Pts',(-2.13439228826135,-2.77524684250714,
-9.65556757699222));
#30142=CARTESIAN_POINT('Ctrl Pts',(-2.07514372551651,2.15791220141318,-9.8120026091365));
#30143=CARTESIAN_POINT('Ctrl Pts',(-2.01589516277168,6.57024637957694,-7.60025281042448));
#30144=CARTESIAN_POINT('Ctrl Pts',(-1.95664660002684,9.39681275570056,-3.554137068968));
#30145=CARTESIAN_POINT('Ctrl Pts',(-1.89739803728201,9.95540282638318,1.34979066345517));
#30146=CARTESIAN_POINT('Ctrl Pts',(-1.83814947453718,8.11119757610343,5.92793844031152));
#30147=CARTESIAN_POINT('Ctrl Pts',(-1.77890091179234,4.30930684356341,9.07534323310842));
#30148=CARTESIAN_POINT('Ctrl Pts',(-1.71965234904751,-0.532660569034724,
10.0323602900267));
#30149=CARTESIAN_POINT('Ctrl Pts',(-1.66040378630267,-5.24606720460977,
8.56800788721785));
#30150=CARTESIAN_POINT('Ctrl Pts',(-1.60115522355784,-8.6933045095691,5.03571613324405));
#30151=CARTESIAN_POINT('Ctrl Pts',(-1.541906660813,-10.0423613829002,0.288024523165256));
#30152=CARTESIAN_POINT('Ctrl Pts',(-1.48265809806817,-8.96763497362019,
-4.52918350816273));
#30153=CARTESIAN_POINT('Ctrl Pts',(-1.42340953532333,-5.72851685357889,
-8.25324632668694));
#30154=CARTESIAN_POINT('Ctrl Pts',(-1.3641609725785,-1.10678732826568,-9.98533935731279));
#30155=CARTESIAN_POINT('Ctrl Pts',(-1.30491240983366,3.78207186121437,-9.3074117082742));
#30156=CARTESIAN_POINT('Ctrl Pts',(-1.24566384708883,7.75810565024088,-6.38308522506237));
#30157=CARTESIAN_POINT('Ctrl Pts',(-1.18641528434399,9.86167478052657,-1.91816339080776));
#30158=CARTESIAN_POINT('Ctrl Pts',(-1.12716672159916,9.58507040776671,3.00971851655006));
#30159=CARTESIAN_POINT('Ctrl Pts',(-1.06791815885432,6.99505263240274,7.21118706875814));
#30160=CARTESIAN_POINT('Ctrl Pts',(-1.00866959610949,2.71673755474579,9.67219299483537));
#30161=CARTESIAN_POINT('Ctrl Pts',(-0.949421033364656,-2.21727819104757,
9.79875796691677));
#30162=CARTESIAN_POINT('Ctrl Pts',(-0.890172470619816,-6.61614073855928,
7.56033478083375));
#30163=CARTESIAN_POINT('Ctrl Pts',(-0.830923907874984,-9.41815860919774,
3.49718010441341));
#30164=CARTESIAN_POINT('Ctrl Pts',(-0.771675345130147,-9.94704822647297,
-1.41003966289232));
#30165=CARTESIAN_POINT('Ctrl Pts',(-0.712426782385315,-8.07515895486045,
-5.9769380224696));
#30166=CARTESIAN_POINT('Ctrl Pts',(-0.653178219640479,-4.25428233525734,
-9.1012670591868));
#30167=CARTESIAN_POINT('Ctrl Pts',(-0.593929656895646,0.593390474060013,
-10.0289514913561));
#30168=CARTESIAN_POINT('Ctrl Pts',(-0.534681094150809,5.29784498478896,
-8.53608919751393));
#30169=CARTESIAN_POINT('Ctrl Pts',(-0.475432531405974,8.72363329158144,
-4.98299131693383));
#30170=CARTESIAN_POINT('Ctrl Pts',(-0.416183968661139,10.0439211359327,
-0.227219026357994));
#30171=CARTESIAN_POINT('Ctrl Pts',(-0.356935405916306,8.94004924204562,
4.58339391942193));
#30172=CARTESIAN_POINT('Ctrl Pts',(-0.297686843171469,5.67844361680366,
8.28777764910186));
#30173=CARTESIAN_POINT('Ctrl Pts',(-0.238438280426636,1.04631205793237,
9.99185725226522));
#30174=CARTESIAN_POINT('Ctrl Pts',(-0.179189717681799,-3.83835310103361,
9.28434304296069));
#30175=CARTESIAN_POINT('Ctrl Pts',(-0.119941154936966,-7.79660904980335,
6.335997758854));
#30176=CARTESIAN_POINT('Ctrl Pts',(-0.0606925921921299,-9.87310731639768,
1.8584219607967));
#30177=CARTESIAN_POINT('Ctrl Pts',(-0.00144402944729562,-9.56667277050388,
-3.06769496072332));
#30178=CARTESIAN_POINT('Ctrl Pts',(0.0578045332975387,-6.95126519921767,
-7.25340557413907));
#30179=CARTESIAN_POINT('Ctrl Pts',(0.117053096042374,-2.65812868397592,
-9.68846386678141));
#30180=CARTESIAN_POINT('Ctrl Pts',(0.176301658787208,2.27656290681844,-9.78515415130587));
#30181=CARTESIAN_POINT('Ctrl Pts',(0.235550221532044,6.6617925734103,-7.52013960614428));
#30182=CARTESIAN_POINT('Ctrl Pts',(0.294798784276878,9.43915924093234,-3.44009497706739));
#30183=CARTESIAN_POINT('Ctrl Pts',(0.354047347021712,9.93832899371509,1.47023703241122));
#30184=CARTESIAN_POINT('Ctrl Pts',(0.413295909766548,8.03882436311626,6.02571840673295));
#30185=CARTESIAN_POINT('Ctrl Pts',(0.472544472511384,4.19910182337586,9.12685748071474));
#30186=CARTESIAN_POINT('Ctrl Pts',(0.531793035256219,-0.654098512982282,
10.0251746688745));
#30187=CARTESIAN_POINT('Ctrl Pts',(0.591041598001053,-5.34942879018335,
8.50385839223102));
#30188=CARTESIAN_POINT('Ctrl Pts',(0.650290160745887,-8.75364187343509,
4.9300823360043));
#30189=CARTESIAN_POINT('Ctrl Pts',(0.709538723490721,-10.0451135486074,
0.166408114964229));
#30190=CARTESIAN_POINT('Ctrl Pts',(0.768787286235557,-8.91213420796575,
-4.637441950575));
#30191=CARTESIAN_POINT('Ctrl Pts',(0.828035848980392,-5.62816531801462,
-8.32199430859616));
#30192=CARTESIAN_POINT('Ctrl Pts',(0.887284411725228,-0.985792475144742,
-9.99802987535393));
#30193=CARTESIAN_POINT('Ctrl Pts',(0.946532974470062,3.89448213486398,-9.26089351818321));
#30194=CARTESIAN_POINT('Ctrl Pts',(1.0057815372149,7.83484888772788,-6.28875637178055));
#30195=CARTESIAN_POINT('Ctrl Pts',(1.06503009995973,9.88413496211296,-1.79846062562306));
#30196=CARTESIAN_POINT('Ctrl Pts',(1.12427866270457,9.54800801276635,3.12526083781895));
#30197=CARTESIAN_POINT('Ctrl Pts',(1.1835272254494,6.90705632238448,7.29598208910701));
#30198=CARTESIAN_POINT('Ctrl Pts',(1.22302626727929,4.03555160320576,8.90048051538159));
#30199=CARTESIAN_POINT('Ctrl Pts',(1.24277578819424,2.49464822519328,9.31322804590546));
#30200=CARTESIAN_POINT('Ctrl Pts',(-8.08092526273141,7.32294389040362,-6.48509627723018));
#30201=CARTESIAN_POINT('Ctrl Pts',(-8.06117574181647,8.39592381863735,-5.27349178069048));
#30202=CARTESIAN_POINT('Ctrl Pts',(-8.02167669998657,9.92797148557023,-2.30875446498139));
#30203=CARTESIAN_POINT('Ctrl Pts',(-7.96242813724176,9.82880183853739,2.69858166596329));
#30204=CARTESIAN_POINT('Ctrl Pts',(-7.9031795744969,7.35781851876972,7.05329954423695));
#30205=CARTESIAN_POINT('Ctrl Pts',(-7.84393101175208,3.11077563954764,9.70630784040932));
#30206=CARTESIAN_POINT('Ctrl Pts',(-7.78468244900724,-1.88696580672517,
10.0163096700013));
#30207=CARTESIAN_POINT('Ctrl Pts',(-7.7254338862624,-6.42933139469688,7.90898742424441));
#30208=CARTESIAN_POINT('Ctrl Pts',(-7.66618532351757,-9.41991164186956,
3.89269554661848));
#30209=CARTESIAN_POINT('Ctrl Pts',(-7.60693676077273,-10.1369551341012,
-1.06307544883298));
#30210=CARTESIAN_POINT('Ctrl Pts',(-7.5476881980279,-8.40737702072891,-5.76229070180903));
#30211=CARTESIAN_POINT('Ctrl Pts',(-7.48843963528306,-4.64863268122753,
-9.07073070640136));
#30212=CARTESIAN_POINT('Ctrl Pts',(-7.42919107253823,0.23208866289055,-10.1899026181865));
#30213=CARTESIAN_POINT('Ctrl Pts',(-7.36994250979339,5.05679298620976,-8.84967799296175));
#30214=CARTESIAN_POINT('Ctrl Pts',(-7.31069394704856,8.66101097414312,-5.37353298305073));
#30215=CARTESIAN_POINT('Ctrl Pts',(-7.25144538430373,10.1748424845305,-0.600453137120963));
#30216=CARTESIAN_POINT('Ctrl Pts',(-7.19219682155888,9.23291576111782,4.31754916391827));
#30217=CARTESIAN_POINT('Ctrl Pts',(-7.13294825881406,6.06257016523153,8.19348568982741));
#30218=CARTESIAN_POINT('Ctrl Pts',(-7.07369969606921,1.42898746173764,10.0918758877297));
#30219=CARTESIAN_POINT('Ctrl Pts',(-7.01445113332439,-3.54948983298891,
9.55453224832087));
#30220=CARTESIAN_POINT('Ctrl Pts',(-6.95520257057954,-7.67127676413759,
6.71114573860529));
#30221=CARTESIAN_POINT('Ctrl Pts',(-6.89595400783472,-9.94155570690313,
2.24798455074812));
#30222=CARTESIAN_POINT('Ctrl Pts',(-6.83670544508988,-9.81238141003462,
-2.7577410056674));
#30223=CARTESIAN_POINT('Ctrl Pts',(-6.77745688234504,-7.31493085792997,
-7.09786946410221));
#30224=CARTESIAN_POINT('Ctrl Pts',(-6.71820831960022,-3.05197850216906,
-9.72488517251122));
#30225=CARTESIAN_POINT('Ctrl Pts',(-6.65895975685537,1.94758690568939,-10.0047423571369));
#30226=CARTESIAN_POINT('Ctrl Pts',(-6.59971119411055,6.47709070140057,-7.8698958340312));
#30227=CARTESIAN_POINT('Ctrl Pts',(-6.5404626313657,9.44331036856071,-3.83560343017826));
#30228=CARTESIAN_POINT('Ctrl Pts',(-6.48121406862087,10.1303312566116,1.12443453456516));
#30229=CARTESIAN_POINT('Ctrl Pts',(-6.42196550587604,8.37233681299167,5.8130835776728));
#30230=CARTESIAN_POINT('Ctrl Pts',(-6.3627169431312,4.59362938864533,9.09871053670815));
#30231=CARTESIAN_POINT('Ctrl Pts',(-6.30346838038637,-0.293777642722069,
10.188309923035));
#30232=CARTESIAN_POINT('Ctrl Pts',(-6.24421981764153,-5.11027970342329,
8.8189004838395));
#30233=CARTESIAN_POINT('Ctrl Pts',(-6.1849712548967,-8.69338554959525,5.32099728220349));
#30234=CARTESIAN_POINT('Ctrl Pts',(-6.12572269215187,-10.1782914046486,
0.538839932791344));
#30235=CARTESIAN_POINT('Ctrl Pts',(-6.06647412940702,-9.20660646282684,
-4.37336961961261));
#30236=CARTESIAN_POINT('Ctrl Pts',(-6.0072255666622,-6.01285262870474,-8.23004056226918));
#30237=CARTESIAN_POINT('Ctrl Pts',(-5.94797700391735,-1.36786126920608,
-10.1003425654441));
#30238=CARTESIAN_POINT('Ctrl Pts',(-5.88872844117253,3.60727149337718,-9.53286718486024));
#30239=CARTESIAN_POINT('Ctrl Pts',(-5.82947987842769,7.711767957572,-6.6645779581067));
#30240=CARTESIAN_POINT('Ctrl Pts',(-5.77023131568285,9.95498363906506,-2.18775344521796));
#30241=CARTESIAN_POINT('Ctrl Pts',(-5.71098275293802,9.79550517293285,2.8170982940185));
#30242=CARTESIAN_POINT('Ctrl Pts',(-5.65173419019318,7.27182362969249,7.14202670743828));
#30243=CARTESIAN_POINT('Ctrl Pts',(-5.59248562744835,2.99304446790236,9.74318475675563));
#30244=CARTESIAN_POINT('Ctrl Pts',(-5.53323706470351,-2.0081236688321,9.99276757068793));
#30245=CARTESIAN_POINT('Ctrl Pts',(-5.47398850195868,-6.524619287585,7.83053686174773));
#30246=CARTESIAN_POINT('Ctrl Pts',(-5.41473993921384,-9.46635947266288,
3.77835979301097));
#30247=CARTESIAN_POINT('Ctrl Pts',(-5.35549137646901,-10.1233378410533,
-1.18574674657548));
#30248=CARTESIAN_POINT('Ctrl Pts',(-5.29624281372418,-8.33698877998584,
-5.86366629963766));
#30249=CARTESIAN_POINT('Ctrl Pts',(-5.23699425097934,-4.5384581948942,-9.12635532972027));
#30250=CARTESIAN_POINT('Ctrl Pts',(-5.17774568823451,0.355456103468731,
-10.1863445528621));
#30251=CARTESIAN_POINT('Ctrl Pts',(-5.11849712548966,5.16357897007176,-8.78779930420289));
#30252=CARTESIAN_POINT('Ctrl Pts',(-5.05924856274484,8.72544152907295,-5.26826674664877));
#30253=CARTESIAN_POINT('Ctrl Pts',(-5.,10.1813671968188,-0.477206867780972));
#30254=CARTESIAN_POINT('Ctrl Pts',(-4.94075143725517,9.17995970706714,4.429029709512));
#30255=CARTESIAN_POINT('Ctrl Pts',(-4.88150287451032,5.96291467703338,8.26629378533911));
#30256=CARTESIAN_POINT('Ctrl Pts',(-4.82225431176551,1.30668494145425,10.1084389919954));
#30257=CARTESIAN_POINT('Ctrl Pts',(-4.76300574902065,-3.66492092887833,
9.51085269448463));
#30258=CARTESIAN_POINT('Ctrl Pts',(-4.70375718627583,-7.75197646878442,
6.61776587818947));
#30259=CARTESIAN_POINT('Ctrl Pts',(-4.64450862353099,-9.9680466641253,2.12744214796467));
#30260=CARTESIAN_POINT('Ctrl Pts',(-4.58526006078616,-9.77826987352389,
-2.87635232050094));
#30261=CARTESIAN_POINT('Ctrl Pts',(-4.52601149804132,-7.22844984720876,
-7.18592215359337));
#30262=CARTESIAN_POINT('Ctrl Pts',(-4.46676293529649,-2.93400072113927,
-9.76112719717709));
#30263=CARTESIAN_POINT('Ctrl Pts',(-4.40751437255165,2.06858682257122,-9.98042649131794));
#30264=CARTESIAN_POINT('Ctrl Pts',(-4.34826580980682,6.5719087087328,-7.79089085504336));
#30265=CARTESIAN_POINT('Ctrl Pts',(-4.28901724706198,9.48906157988604,-3.72097765704751));
#30266=CARTESIAN_POINT('Ctrl Pts',(-4.22976868431715,10.1159733465758,1.24701549408342));
#30267=CARTESIAN_POINT('Ctrl Pts',(-4.17052012157231,8.30133514808314,5.91403408430452));
#30268=CARTESIAN_POINT('Ctrl Pts',(-4.11127155882748,4.48312064038335,9.15366558898046));
#30269=CARTESIAN_POINT('Ctrl Pts',(-4.05202299608264,-0.417121534692773,
10.1840057942055));
#30270=CARTESIAN_POINT('Ctrl Pts',(-3.99277443333782,-5.21668896166365,
8.75637600085633));
#30271=CARTESIAN_POINT('Ctrl Pts',(-3.93352587059297,-8.75717767061589,
5.2153430986257));
#30272=CARTESIAN_POINT('Ctrl Pts',(-3.87427730784814,-10.1840697829513,
0.415556310376332));
#30273=CARTESIAN_POINT('Ctrl Pts',(-3.8150287451033,-9.15297645265046,-4.48452744983706));
#30274=CARTESIAN_POINT('Ctrl Pts',(-3.75578018235847,-5.91275815002565,
-8.30224400089647));
#30275=CARTESIAN_POINT('Ctrl Pts',(-3.69653161961363,-1.24546071613625,
-10.1161648857498));
#30276=CARTESIAN_POINT('Ctrl Pts',(-3.6372830568688,3.72243602381481,-9.48848957630887));
#30277=CARTESIAN_POINT('Ctrl Pts',(-3.57803449412397,7.79190082519069,-6.57071121884904));
#30278=CARTESIAN_POINT('Ctrl Pts',(-3.51878593137913,9.9807443025801,-2.06705286764298));
#30279=CARTESIAN_POINT('Ctrl Pts',(-3.4595373686343,9.76067614392728,2.93550091202248));
#30280=CARTESIAN_POINT('Ctrl Pts',(-3.40028880588946,7.18481110019973,7.22955419410927));
#30281=CARTESIAN_POINT('Ctrl Pts',(-3.34104024314463,2.8748494262677,9.77871183578925));
#30282=CARTESIAN_POINT('Ctrl Pts',(-3.28179168039979,-2.12897415063036,
9.96771957155015));
#30283=CARTESIAN_POINT('Ctrl Pts',(-3.22254311765496,-6.61895723138814,
7.7509592670953));
#30284=CARTESIAN_POINT('Ctrl Pts',(-3.16329455491012,-9.51141585807944,
3.66345912571588));
#30285=CARTESIAN_POINT('Ctrl Pts',(-3.10404599216529,-10.1082380431237,
-1.30823853125571));
#30286=CARTESIAN_POINT('Ctrl Pts',(-3.04479742942045,-8.26537722419904,
-5.96418508539163));
#30287=CARTESIAN_POINT('Ctrl Pts',(-2.98554886667561,-4.42761875355267,
-9.18064031341523));
#30288=CARTESIAN_POINT('Ctrl Pts',(-2.92630030393078,0.478771675998264,
-10.1812937327914));
#30289=CARTESIAN_POINT('Ctrl Pts',(-2.86705174118595,5.26960773141081,-8.72463172564731));
#30290=CARTESIAN_POINT('Ctrl Pts',(-2.80780317844111,8.78859281091049,-5.16222827809161));
#30291=CARTESIAN_POINT('Ctrl Pts',(-2.74855461569627,10.1863990639807,-0.353890520427748));
#30292=CARTESIAN_POINT('Ctrl Pts',(-2.68930605295144,9.12565768866926,4.53986080627456));
#30293=CARTESIAN_POINT('Ctrl Pts',(-2.63005749020661,5.86238488620854,8.33788989115769));
#30294=CARTESIAN_POINT('Ctrl Pts',(-2.57080892746177,1.18419083747417,10.1235199635087));
#30295=CARTESIAN_POINT('Ctrl Pts',(-2.51156036471694,-3.77981466992552,
9.46577865007057));
#30296=CARTESIAN_POINT('Ctrl Pts',(-2.4523118019721,-7.83153956333209,6.52341570491109));
#30297=CARTESIAN_POINT('Ctrl Pts',(-2.39306323922726,-9.99307608898748,
2.00658781786958));
#30298=CARTESIAN_POINT('Ctrl Pts',(-2.33381467648243,-9.74272462905507,
-2.99454190044487));
#30299=CARTESIAN_POINT('Ctrl Pts',(-2.2745661137376,-7.14090898827806,-7.2729212296192));
#30300=CARTESIAN_POINT('Ctrl Pts',(-2.21531755099276,-2.81559275152503,
-9.79593802801323));
#30301=CARTESIAN_POINT('Ctrl Pts',(-2.15606898824792,2.18928343946426,-9.95464727716678));
#30302=CARTESIAN_POINT('Ctrl Pts',(-2.0968204255031,6.66576313095033,-7.71074356162747));
#30303=CARTESIAN_POINT('Ctrl Pts',(-2.03757186275825,9.53342148782944,-3.60580630740307));
#30304=CARTESIAN_POINT('Ctrl Pts',(-1.97832330001343,10.1001322142407,1.36941361391379));
#30305=CARTESIAN_POINT('Ctrl Pts',(-1.91907473726858,8.2291163263995,6.0141174645746));
#30306=CARTESIAN_POINT('Ctrl Pts',(-1.85982617452376,4.37195456886755,9.20727851424482));
#30307=CARTESIAN_POINT('Ctrl Pts',(-1.80057761177892,-0.540404267550662,
10.1782084680325));
#30308=CARTESIAN_POINT('Ctrl Pts',(-1.74132904903408,-5.32233333953408,
8.69256764218722));
#30309=CARTESIAN_POINT('Ctrl Pts',(-1.68208048628925,-8.81968579841007,
5.10892423201202));
#30310=CARTESIAN_POINT('Ctrl Pts',(-1.62283192354441,-10.1883549545254,
0.292211758343243));
#30311=CARTESIAN_POINT('Ctrl Pts',(-1.56358336079958,-9.09800441651432,
-4.59502775053671));
#30312=CARTESIAN_POINT('Ctrl Pts',(-1.50433479805474,-5.81179673205382,
-8.37323014949454));
#30313=CARTESIAN_POINT('Ctrl Pts',(-1.44508623530991,-1.12287755136383,
-10.1305039556658));
#30314=CARTESIAN_POINT('Ctrl Pts',(-1.38583767256507,3.83705476395099,-9.44272074825668));
#30315=CARTESIAN_POINT('Ctrl Pts',(-1.32658910982024,7.87089123021942,-6.47588107002986));
#30316=CARTESIAN_POINT('Ctrl Pts',(-1.2673405470754,10.0050415713161,-1.94604921503846));
#30317=CARTESIAN_POINT('Ctrl Pts',(-1.20809198433057,9.72441598693415,3.05347312157412));
#30318=CARTESIAN_POINT('Ctrl Pts',(-1.14884342158573,7.09674512071032,7.31602167047027));
#30319=CARTESIAN_POINT('Ctrl Pts',(-1.0895948588409,2.75623286901131,9.81280514240945));
#30320=CARTESIAN_POINT('Ctrl Pts',(-1.03034629609607,-2.24951247838848,
9.94121008734307));
#30321=CARTESIAN_POINT('Ctrl Pts',(-0.97109773335123,-6.71232469171219,
7.67024521277815));
#30322=CARTESIAN_POINT('Ctrl Pts',(-0.911849170606395,-9.55507766250236,
3.54802131541876));
#30323=CARTESIAN_POINT('Ctrl Pts',(-0.85260060786156,-10.0916561570523,
-1.43053849963697));
#30324=CARTESIAN_POINT('Ctrl Pts',(-0.793352045116725,-8.19255378385643,
-6.06382939154229));
#30325=CARTESIAN_POINT('Ctrl Pts',(-0.734103482371892,-4.31613012674232,
-9.23357921502578));
#30326=CARTESIAN_POINT('Ctrl Pts',(-0.674854919627057,0.602017050158339,
-10.1747501130201));
#30327=CARTESIAN_POINT('Ctrl Pts',(-0.615606356882222,5.37486385333546,
-8.66018492581331));
#30328=CARTESIAN_POINT('Ctrl Pts',(-0.556357794137386,8.85045549337507,
-5.05543291428316));
#30329=CARTESIAN_POINT('Ctrl Pts',(-0.497109231392552,10.1899373828937,
-0.230522285017434));
#30330=CARTESIAN_POINT('Ctrl Pts',(-0.437860668647717,9.07001764983207,
4.65002626045691));
#30331=CARTESIAN_POINT('Ctrl Pts',(-0.378612105902882,5.76099554192171,
8.40826348044112));
#30332=CARTESIAN_POINT('Ctrl Pts',(-0.319363543158047,1.06152310526953,
10.1371166062964));
#30333=CARTESIAN_POINT('Ctrl Pts',(-0.260114980413212,-3.89415420766704,
9.41931671592008));
#30334=CARTESIAN_POINT('Ctrl Pts',(-0.200866417668378,-7.90995438347004,
6.42810905691977));
#30335=CARTESIAN_POINT('Ctrl Pts',(-0.141617854923542,-10.0166403108002,
1.88543927767054));
#30336=CARTESIAN_POINT('Ctrl Pts',(-0.0823692921787074,-9.7057508889944,
-3.11229241414054));
#30337=CARTESIAN_POINT('Ctrl Pts',(-0.0231207294338736,-7.05232111575499,
-7.35885393890494));
#30338=CARTESIAN_POINT('Ctrl Pts',(0.0361278333109621,-2.69677195577391,
-9.82931255660071));
#30339=CARTESIAN_POINT('Ctrl Pts',(0.0953763960557961,2.3096590619082,-9.9274085025469));
#30340=CARTESIAN_POINT('Ctrl Pts',(0.154624958800632,6.75864020258194,-7.62946568975753));
#30341=CARTESIAN_POINT('Ctrl Pts',(0.213873521545465,9.57638359665701,-3.49010629744142));
#30342=CARTESIAN_POINT('Ctrl Pts',(0.273122084290301,10.0828101660666,1.49161100485786));
#30343=CARTESIAN_POINT('Ctrl Pts',(0.332370647035135,8.15569096806016,6.11331893396601));
#30344=CARTESIAN_POINT('Ctrl Pts',(0.391619209779972,4.26014741309707,9.25954166429657));
#30345=CARTESIAN_POINT('Ctrl Pts',(0.450867772524807,-0.663607648778533,
10.1709183839501));
#30346=CARTESIAN_POINT('Ctrl Pts',(0.510116335269641,-5.42719757239065,
8.62748555639489));
#30347=CARTESIAN_POINT('Ctrl Pts',(0.569364898014475,-8.8809003331841,5.00175475459157));
#30348=CARTESIAN_POINT('Ctrl Pts',(0.628613460759309,-10.1911471305933,
0.168827318389068));
#30349=CARTESIAN_POINT('Ctrl Pts',(0.687862023504144,-9.04169679331941,
-4.7048600296258));
#30350=CARTESIAN_POINT('Ctrl Pts',(0.747110586248981,-5.70998630863076,
-8.44297757396894));
#30351=CARTESIAN_POINT('Ctrl Pts',(0.806359148993815,-1.0001237025165,-10.1433789655793));
#30352=CARTESIAN_POINT('Ctrl Pts',(0.865607711738651,3.95109923265809,-9.39552628727104));
#30353=CARTESIAN_POINT('Ctrl Pts',(0.924856274483485,7.94875014348341,-6.38018088527799));
#30354=CARTESIAN_POINT('Ctrl Pts',(0.984104837228319,10.0278282739272,-1.82460623820867));
#30355=CARTESIAN_POINT('Ctrl Pts',(1.04335339997315,9.68681478724308,3.17069517089827));
#30356=CARTESIAN_POINT('Ctrl Pts',(1.10260196271799,7.0074695402994,7.40204942158881));
#30357=CARTESIAN_POINT('Ctrl Pts',(1.14210100454788,4.09421953692831,9.02987368199615));
#30358=CARTESIAN_POINT('Ctrl Pts',(1.16185052546282,2.53091485516785,9.44862164248496));
#30359=CARTESIAN_POINT('Ctrl Pts',(-8.16185052546282,7.42787768375328,-6.57802417109255));
#30360=CARTESIAN_POINT('Ctrl Pts',(-8.14210100454788,8.51623282935078,-5.34905804270585));
#30361=CARTESIAN_POINT('Ctrl Pts',(-8.102601962718,10.070233904051,-2.34183765769039));
#30362=CARTESIAN_POINT('Ctrl Pts',(-8.04335339997314,9.96964321004528,2.73725086992161));
#30363=CARTESIAN_POINT('Ctrl Pts',(-7.98410483722833,7.4632520465296,7.15436948112095));
#30364=CARTESIAN_POINT('Ctrl Pts',(-7.92485627448348,3.15535135841191,9.84539393970996));
#30365=CARTESIAN_POINT('Ctrl Pts',(-7.86560771173865,-1.91400499792807,
10.1598379265015));
#30366=CARTESIAN_POINT('Ctrl Pts',(-7.80635914899382,-6.52146020819656,
8.0223189019126));
#30367=CARTESIAN_POINT('Ctrl Pts',(-7.74711058624898,-9.55489383979345,
3.94847575143437));
#30368=CARTESIAN_POINT('Ctrl Pts',(-7.68786202350415,-10.2822121743239,
-1.07830874040703));
#30369=CARTESIAN_POINT('Ctrl Pts',(-7.62861346075931,-8.5278501495838,-5.84486118586212));
#30370=CARTESIAN_POINT('Ctrl Pts',(-7.56936489801448,-4.71524505303195,
-9.20070933189968));
#30371=CARTESIAN_POINT('Ctrl Pts',(-7.51011633526964,0.23541436689089,-10.3359183669881));
#30372=CARTESIAN_POINT('Ctrl Pts',(-7.4508677725248,5.12925407264827,-8.97648905359836));
#30373=CARTESIAN_POINT('Ctrl Pts',(-7.39161920977998,8.78511853926469,-5.45053278095167));
#30374=CARTESIAN_POINT('Ctrl Pts',(-7.33237064703513,10.3206424298279,-0.609057303198129));
#30375=CARTESIAN_POINT('Ctrl Pts',(-7.27312208429031,9.36521841002403,4.37941728943228));
#30376=CARTESIAN_POINT('Ctrl Pts',(-7.21387352154547,6.14944349027773,8.31089387252787));
#30377=CARTESIAN_POINT('Ctrl Pts',(-7.15462495880063,1.44946407295485,10.2364869669299));
#30378=CARTESIAN_POINT('Ctrl Pts',(-7.0953763960558,-3.60035208705037,9.69144348613765));
#30379=CARTESIAN_POINT('Ctrl Pts',(-7.03612783331096,-7.78120197765055,
6.80731279800296));
#30380=CARTESIAN_POINT('Ctrl Pts',(-6.97687927056613,-10.0840127798693,
2.280196943719));
#30381=CARTESIAN_POINT('Ctrl Pts',(-6.91763070782129,-9.95298748575479,
-2.79725793070895));
#30382=CARTESIAN_POINT('Ctrl Pts',(-6.85838214507646,-7.41974982889312,
-7.19957806363757));
#30383=CARTESIAN_POINT('Ctrl Pts',(-6.79913358233162,-3.09571169011194,
-9.86423747485219));
#30384=CARTESIAN_POINT('Ctrl Pts',(-6.73988501958679,1.97549476418875,-10.1481048603504));
#30385=CARTESIAN_POINT('Ctrl Pts',(-6.68063645684196,6.56990387972609,-7.98266715052507));
#30386=CARTESIAN_POINT('Ctrl Pts',(-6.62138789409711,9.57862785748067,-3.8905655360932));
#30387=CARTESIAN_POINT('Ctrl Pts',(-6.56213933135229,10.2754933802813,1.14054706838368));
#30388=CARTESIAN_POINT('Ctrl Pts',(-6.50289076860745,8.49230783477424,5.89638189594384));
#30389=CARTESIAN_POINT('Ctrl Pts',(-6.44364220586261,4.65945359325582,9.22909009791965));
#30390=CARTESIAN_POINT('Ctrl Pts',(-6.38439364311778,-0.297987316169458,
10.3343028493835));
#30391=CARTESIAN_POINT('Ctrl Pts',(-6.32514508037294,-5.18350722535756,
8.94527051955084));
#30392=CARTESIAN_POINT('Ctrl Pts',(-6.26589651762811,-8.81795702473186,
5.3972442721547));
#30393=CARTESIAN_POINT('Ctrl Pts',(-6.20664795488328,-10.3241407710909,
0.546561215243084));
#30394=CARTESIAN_POINT('Ctrl Pts',(-6.14739939213844,-9.33853211383284,
-4.43603762182241));
#30395=CARTESIAN_POINT('Ctrl Pts',(-6.08815082939361,-6.09901352855942,
-8.34797255636136));
#30396=CARTESIAN_POINT('Ctrl Pts',(-6.02890226664877,-1.38746197541141,
-10.2450749675197));
#30397=CARTESIAN_POINT('Ctrl Pts',(-5.96965370390394,3.65896172712842,-9.6694679741298));
#30398=CARTESIAN_POINT('Ctrl Pts',(-5.9104051411591,7.82227338781035,-6.76007772659941));
#30399=CARTESIAN_POINT('Ctrl Pts',(-5.85115657841427,10.097633126978,-2.21910275928568));
#30400=CARTESIAN_POINT('Ctrl Pts',(-5.79190801566943,9.93586942137656,2.85746577663947));
#30401=CARTESIAN_POINT('Ctrl Pts',(-5.7326594529246,7.37602489757785,7.24436805619533));
#30402=CARTESIAN_POINT('Ctrl Pts',(-5.67341089017976,3.03593316326608,9.88279928216156));
#30403=CARTESIAN_POINT('Ctrl Pts',(-5.61416232743494,-2.03689898614156,
10.1359584817405));
#30404=CARTESIAN_POINT('Ctrl Pts',(-5.55491376469008,-6.61811352463711,
7.94274418562801));
#30405=CARTESIAN_POINT('Ctrl Pts',(-5.49566520194526,-9.60200724267784,
3.83250162881555));
#30406=CARTESIAN_POINT('Ctrl Pts',(-5.43641663920042,-10.268399752891,-1.2027378509636));
#30407=CARTESIAN_POINT('Ctrl Pts',(-5.37716807645559,-8.45645328372782,
-5.94768944073586));
#30408=CARTESIAN_POINT('Ctrl Pts',(-5.31791951371075,-4.60349182637855,
-9.2571310257432));
#30409=CARTESIAN_POINT('Ctrl Pts',(-5.25867095096592,0.360549595630422,
-10.3323093165276));
#30410=CARTESIAN_POINT('Ctrl Pts',(-5.19942238822108,5.23757024143739,-8.91372367696696));
#30411=CARTESIAN_POINT('Ctrl Pts',(-5.14017382547626,8.85047234891796,-5.3437581367751));
#30412=CARTESIAN_POINT('Ctrl Pts',(-5.0809252627314,10.327260637686,-0.484044982014571));
#30413=CARTESIAN_POINT('Ctrl Pts',(-5.02167669998659,9.31150352459139,4.49249529046319));
#30414=CARTESIAN_POINT('Ctrl Pts',(-4.96242813724174,6.04835999326767,8.38474526835198));
#30415=CARTESIAN_POINT('Ctrl Pts',(-4.90317957449691,1.32540902423731,10.2532874114492));
#30416=CARTESIAN_POINT('Ctrl Pts',(-4.84393101175207,-3.7174372476088,9.64713802810981));
#30417=CARTESIAN_POINT('Ctrl Pts',(-4.78468244900724,-7.86305806506605,
6.71259485509974));
#30418=CARTESIAN_POINT('Ctrl Pts',(-4.7254338862624,-10.1108833380651,2.15792723402554));
#30419=CARTESIAN_POINT('Ctrl Pts',(-4.66618532351757,-9.91838714952408,
-2.91756888101505));
#30420=CARTESIAN_POINT('Ctrl Pts',(-4.60693676077273,-7.33202959243926,
-7.28889250016123));
#30421=CARTESIAN_POINT('Ctrl Pts',(-4.5476881980279,-2.97604335180359,-9.90099882797171));
#30422=CARTESIAN_POINT('Ctrl Pts',(-4.48843963528306,2.09822854390817,-10.1234405614317));
#30423=CARTESIAN_POINT('Ctrl Pts',(-4.42919107253823,6.66608057740692,-7.90253007326325));
#30424=CARTESIAN_POINT('Ctrl Pts',(-4.36994250979339,9.62503465871992,-3.77429723812952));
#30425=CARTESIAN_POINT('Ctrl Pts',(-4.31069394704856,10.2609297292228,1.26488454621852));
#30426=CARTESIAN_POINT('Ctrl Pts',(-4.25144538430372,8.42028875471895,5.99877896829557));
#30427=CARTESIAN_POINT('Ctrl Pts',(-4.19219682155889,4.54736131488258,9.28483262612855));
#30428=CARTESIAN_POINT('Ctrl Pts',(-4.13294825881405,-0.423098658862809,
10.3299370447346));
#30429=CARTESIAN_POINT('Ctrl Pts',(-4.07369969606922,-5.29144127025228,
8.88185009481599));
#30430=CARTESIAN_POINT('Ctrl Pts',(-4.01445113332439,-8.88266325206611,
5.29007612173078));
#30431=CARTESIAN_POINT('Ctrl Pts',(-3.95520257057955,-10.3300019504043,
0.421511005735301));
#30432=CARTESIAN_POINT('Ctrl Pts',(-3.89595400783472,-9.28413361485067,
-4.54878828314875));
#30433=CARTESIAN_POINT('Ctrl Pts',(-3.83670544508988,-5.99748475057414,
-8.42121063089757));
#30434=CARTESIAN_POINT('Ctrl Pts',(-3.77745688234504,-1.26330748915105,
-10.2611240130488));
#30435=CARTESIAN_POINT('Ctrl Pts',(-3.71820831960021,3.77577650249745,-9.62445445864334));
#30436=CARTESIAN_POINT('Ctrl Pts',(-3.65895975685538,7.90355451573215,-6.66486592814603));
#30437=CARTESIAN_POINT('Ctrl Pts',(-3.59971119411054,10.123762926756,-2.09667260824215));
#30438=CARTESIAN_POINT('Ctrl Pts',(-3.5404626313657,9.90054131137476,2.97756503960422));
#30439=CARTESIAN_POINT('Ctrl Pts',(-3.48121406862087,7.28776552597823,7.33314976402877));
#30440=CARTESIAN_POINT('Ctrl Pts',(-3.42196550587603,2.91604445112685,9.91883544486771));
#30441=CARTESIAN_POINT('Ctrl Pts',(-3.3627169431312,-2.15948118945414,10.1105515584317));
#30442=CARTESIAN_POINT('Ctrl Pts',(-3.30346838038637,-6.71380327974022,
7.86202628743132));
#30443=CARTESIAN_POINT('Ctrl Pts',(-3.24421981764153,-9.64770926153188,
3.71595449760403));
#30444=CARTESIAN_POINT('Ctrl Pts',(-3.1849712548967,-10.2530835830897,-1.32698487613358));
#30445=CARTESIAN_POINT('Ctrl Pts',(-3.12572269215186,-8.38381557339049,
-6.04964860588505));
#30446=CARTESIAN_POINT('Ctrl Pts',(-3.06647412940703,-4.49106411627424,
-9.31219388365737));
#30447=CARTESIAN_POINT('Ctrl Pts',(-3.00722556666219,0.485632213080447,
-10.3271861209591));
#30448=CARTESIAN_POINT('Ctrl Pts',(-2.94797700391736,5.34511833711766,-8.84965094145075));
#30449=CARTESIAN_POINT('Ctrl Pts',(-2.88872844117252,8.91452855419303,-5.23620019477759));
#30450=CARTESIAN_POINT('Ctrl Pts',(-2.82947987842769,10.3323646087608,-0.358961578638042));
#30451=CARTESIAN_POINT('Ctrl Pts',(-2.77023131568285,9.2564233878763,4.60491453641526));
#30452=CARTESIAN_POINT('Ctrl Pts',(-2.71098275293802,5.94638966535093,8.45736730733147));
#30453=CARTESIAN_POINT('Ctrl Pts',(-2.65173419019318,1.20115964653319,10.2685844850618));
#30454=CARTESIAN_POINT('Ctrl Pts',(-2.59248562744835,-3.83397735332308,
9.60141809721447));
#30455=CARTESIAN_POINT('Ctrl Pts',(-2.53323706470351,-7.94376125537936,
6.61689269527968));
#30456=CARTESIAN_POINT('Ctrl Pts',(-2.47398850195868,-10.1362714209391,
2.03534112727213));
#30457=CARTESIAN_POINT('Ctrl Pts',(-2.41473993921384,-9.88233256108192,
-3.0374520532005));
#30458=CARTESIAN_POINT('Ctrl Pts',(-2.35549137646901,-7.24323432072894,
-7.37713822551306));
#30459=CARTESIAN_POINT('Ctrl Pts',(-2.29624281372417,-2.85593866054291,
-9.93630847903426));
#30460=CARTESIAN_POINT('Ctrl Pts',(-2.23699425097934,2.22065467751534,-10.097291945197));
#30461=CARTESIAN_POINT('Ctrl Pts',(-2.1777456882345,6.76127988232371,-7.82123431283046));
#30462=CARTESIAN_POINT('Ctrl Pts',(-2.11849712548967,9.67003021995834,-3.65747554583815));
#30463=CARTESIAN_POINT('Ctrl Pts',(-2.05924856274484,10.2448616020983,1.38903656437241));
#30464=CARTESIAN_POINT('Ctrl Pts',(-2.,8.34703507669558,6.10029648883767));
#30465=CARTESIAN_POINT('Ctrl Pts',(-1.94075143725517,4.43460229417169,9.33921379538122));
#30466=CARTESIAN_POINT('Ctrl Pts',(-1.88150287451033,-0.548147966066605,
10.3240566460384));
#30467=CARTESIAN_POINT('Ctrl Pts',(-1.8222543117655,-5.39859947445838,8.8171273971566));
#30468=CARTESIAN_POINT('Ctrl Pts',(-1.76300574902066,-8.94606708725103,
5.18213233078001));
#30469=CARTESIAN_POINT('Ctrl Pts',(-1.70375718627582,-10.3343485261506,
0.296398993521226));
#30470=CARTESIAN_POINT('Ctrl Pts',(-1.64450862353099,-9.22837385940843,
-4.66087199291068));
#30471=CARTESIAN_POINT('Ctrl Pts',(-1.58526006078615,-5.89507661052875,
-8.49321397230215));
#30472=CARTESIAN_POINT('Ctrl Pts',(-1.52601149804132,-1.13896777446197,
-10.2756685540187));
#30473=CARTESIAN_POINT('Ctrl Pts',(-1.46676293529649,3.89203766668761,-9.57802978823917));
#30474=CARTESIAN_POINT('Ctrl Pts',(-1.40751437255165,7.98367681019796,-6.56867691499734));
#30475=CARTESIAN_POINT('Ctrl Pts',(-1.34826580980682,10.1484083621057,-1.97393503926917));
#30476=CARTESIAN_POINT('Ctrl Pts',(-1.28901724706198,9.86376156610162,3.09722772659819));
#30477=CARTESIAN_POINT('Ctrl Pts',(-1.22976868431715,7.19843760901787,7.42085627218239));
#30478=CARTESIAN_POINT('Ctrl Pts',(-1.17052012157231,2.79572818327685,9.95341728998352));
#30479=CARTESIAN_POINT('Ctrl Pts',(-1.11127155882748,-2.2817467657294,10.0836622077694));
#30480=CARTESIAN_POINT('Ctrl Pts',(-1.05202299608264,-6.80850864486509,
7.78015564472256));
#30481=CARTESIAN_POINT('Ctrl Pts',(-0.992774433337806,-9.69199671580699,
3.5988625264241));
#30482=CARTESIAN_POINT('Ctrl Pts',(-0.933525870592972,-10.2362640876317,
-1.45103733638162));
#30483=CARTESIAN_POINT('Ctrl Pts',(-0.874277307848137,-8.30994861285242,
-6.15072076061499));
#30484=CARTESIAN_POINT('Ctrl Pts',(-0.815028745103304,-4.37797791822729,
-9.36589137086476));
#30485=CARTESIAN_POINT('Ctrl Pts',(-0.755780182358469,0.610643626256656,
-10.3205487346842));
#30486=CARTESIAN_POINT('Ctrl Pts',(-0.696531619613634,5.45188272188197,
-8.78428065411268));
#30487=CARTESIAN_POINT('Ctrl Pts',(-0.637283056868798,8.97727769516869,
-5.12787451163251));
#30488=CARTESIAN_POINT('Ctrl Pts',(-0.578034494123964,10.3359536298547,
-0.233825543676864));
#30489=CARTESIAN_POINT('Ctrl Pts',(-0.518785931379129,9.19998605761851,
4.71665860149186));
#30490=CARTESIAN_POINT('Ctrl Pts',(-0.459537368634294,5.84354746703977,
8.52874931178039));
#30491=CARTESIAN_POINT('Ctrl Pts',(-0.400288805889459,1.07673415260668,
10.2823759603276));
#30492=CARTESIAN_POINT('Ctrl Pts',(-0.341040243144623,-3.94995531430047,
9.55429038887948));
#30493=CARTESIAN_POINT('Ctrl Pts',(-0.28179168039979,-8.02329971713674,
6.52022035498553));
#30494=CARTESIAN_POINT('Ctrl Pts',(-0.222543117654954,-10.1601733052027,
1.91245659454439));
#30495=CARTESIAN_POINT('Ctrl Pts',(-0.163294554910119,-9.84482900748493,
-3.15688986755775));
#30496=CARTESIAN_POINT('Ctrl Pts',(-0.104045992165286,-7.1533770322923,
-7.46430230367082));
#30497=CARTESIAN_POINT('Ctrl Pts',(-0.0447974294204499,-2.73541522757191,
-9.97016124642001));
#30498=CARTESIAN_POINT('Ctrl Pts',(0.0144511333243841,2.34275521699797,
-10.0696628537879));
#30499=CARTESIAN_POINT('Ctrl Pts',(0.0736996960692199,6.85548783175356,
-7.73879177337077));
#30500=CARTESIAN_POINT('Ctrl Pts',(0.132948258814054,9.7136079523817,-3.54011761781546));
#30501=CARTESIAN_POINT('Ctrl Pts',(0.192196821558889,10.2272913384181,1.51298497730451));
#30502=CARTESIAN_POINT('Ctrl Pts',(0.251445384303724,8.27255757300405,6.20091946119904));
#30503=CARTESIAN_POINT('Ctrl Pts',(0.31069394704856,4.32119300281829,9.39222584787842));
#30504=CARTESIAN_POINT('Ctrl Pts',(0.369942509793395,-0.673116784574792,
10.3166620990257));
#30505=CARTESIAN_POINT('Ctrl Pts',(0.429191072538228,-5.50496635459793,
8.7511127205588));
#30506=CARTESIAN_POINT('Ctrl Pts',(0.488439635283064,-9.00815879293313,
5.07342717317882));
#30507=CARTESIAN_POINT('Ctrl Pts',(0.547688198027897,-10.3371807125793,
0.171246521813919));
#30508=CARTESIAN_POINT('Ctrl Pts',(0.606936760772733,-9.17125937867306,
-4.77227810867661));
#30509=CARTESIAN_POINT('Ctrl Pts',(0.666185323517568,-5.7918072992469,-8.56396083934171));
#30510=CARTESIAN_POINT('Ctrl Pts',(0.725433886262404,-1.01445492988825,
-10.2887280558046));
#30511=CARTESIAN_POINT('Ctrl Pts',(0.784682449007238,4.0077163304522,-9.53015905635885));
#30512=CARTESIAN_POINT('Ctrl Pts',(0.843931011752074,8.06265139923896,-6.47160539877543));
#30513=CARTESIAN_POINT('Ctrl Pts',(0.903179574496907,10.1715215857415,-1.85075185079428));
#30514=CARTESIAN_POINT('Ctrl Pts',(0.962428137241743,9.8256215617198,3.21612950397759));
#30515=CARTESIAN_POINT('Ctrl Pts',(1.02167669998658,7.10788275821431,7.5081167540706));
#30516=CARTESIAN_POINT('Ctrl Pts',(1.06117574181647,4.15288747065086,9.15926684861071));
#30517=CARTESIAN_POINT('Ctrl Pts',(1.08092526273141,2.56718148514241,9.58401523906446));
#30518=CARTESIAN_POINT('Ctrl Pts',(-8.24277578819424,7.53281147710294,-6.67095206495492));
#30519=CARTESIAN_POINT('Ctrl Pts',(-8.22302626727929,8.6365418400642,-5.42462430472122));
#30520=CARTESIAN_POINT('Ctrl Pts',(-8.1835272254494,10.2124963225319,-2.3749208503994));
#30521=CARTESIAN_POINT('Ctrl Pts',(-8.12427866270457,10.1104845815532,2.77592007387994));
#30522=CARTESIAN_POINT('Ctrl Pts',(-8.06503009995973,7.56868557428947,7.25543941800496));
#30523=CARTESIAN_POINT('Ctrl Pts',(-8.0057815372149,3.19992707727617,9.98448003901059));
#30524=CARTESIAN_POINT('Ctrl Pts',(-7.94653297447006,-1.94104418913098,
10.3033661830017));
#30525=CARTESIAN_POINT('Ctrl Pts',(-7.88728441172523,-6.61358902169624,
8.13565037958078));
#30526=CARTESIAN_POINT('Ctrl Pts',(-7.82803584898039,-9.68987603771733,
4.00425595625027));
#30527=CARTESIAN_POINT('Ctrl Pts',(-7.76878728623556,-10.4274692145465,
-1.09354203198108));
#30528=CARTESIAN_POINT('Ctrl Pts',(-7.70953872349072,-8.64832327843871,
-5.92743166991522));
#30529=CARTESIAN_POINT('Ctrl Pts',(-7.65029016074589,-4.78185742483636,
-9.33068795739798));
#30530=CARTESIAN_POINT('Ctrl Pts',(-7.59104159800105,0.238740070891225,
-10.4819341157898));
#30531=CARTESIAN_POINT('Ctrl Pts',(-7.53179303525622,5.20171515908679,-9.10330011423497));
#30532=CARTESIAN_POINT('Ctrl Pts',(-7.47254447251139,8.90922610438627,-5.52753257885261));
#30533=CARTESIAN_POINT('Ctrl Pts',(-7.41329590976654,10.4664423751253,-0.617661469275298));
#30534=CARTESIAN_POINT('Ctrl Pts',(-7.35404734702172,9.49752105893024,4.4412854149463));
#30535=CARTESIAN_POINT('Ctrl Pts',(-7.29479878427687,6.23631681532395,8.42830205522834));
#30536=CARTESIAN_POINT('Ctrl Pts',(-7.23555022153205,1.46994068417205,10.38109804613));
#30537=CARTESIAN_POINT('Ctrl Pts',(-7.17630165878721,-3.65121434111183,
9.82835472395443));
#30538=CARTESIAN_POINT('Ctrl Pts',(-7.11705309604238,-7.89112719116351,
6.90347985740062));
#30539=CARTESIAN_POINT('Ctrl Pts',(-7.05780453329754,-10.2264698528354,
2.31240933668989));
#30540=CARTESIAN_POINT('Ctrl Pts',(-6.9985559705527,-10.0935935614749,-2.8367748557505));
#30541=CARTESIAN_POINT('Ctrl Pts',(-6.93930740780787,-7.52456879985629,
-7.30128666317293));
#30542=CARTESIAN_POINT('Ctrl Pts',(-6.88005884506304,-3.13944487805482,
-10.0035897771931));
#30543=CARTESIAN_POINT('Ctrl Pts',(-6.8208102823182,2.0034026226881,-10.2914673635639));
#30544=CARTESIAN_POINT('Ctrl Pts',(-6.76156171957337,6.6627170580516,-8.09543846701894));
#30545=CARTESIAN_POINT('Ctrl Pts',(-6.70231315682853,9.71394534640064,-3.94552764200815));
#30546=CARTESIAN_POINT('Ctrl Pts',(-6.6430645940837,10.4206555039509,1.1566596022022));
#30547=CARTESIAN_POINT('Ctrl Pts',(-6.58381603133886,8.61227885655681,5.97968021421488));
#30548=CARTESIAN_POINT('Ctrl Pts',(-6.52456746859403,4.72527779786631,9.35946965913116));
#30549=CARTESIAN_POINT('Ctrl Pts',(-6.46531890584919,-0.302196989616849,
10.480295775732));
#30550=CARTESIAN_POINT('Ctrl Pts',(-6.40607034310435,-5.25673474729183,
9.07164055526217));
#30551=CARTESIAN_POINT('Ctrl Pts',(-6.34682178035952,-8.94252849986846,
5.4734912621059));
#30552=CARTESIAN_POINT('Ctrl Pts',(-6.28757321761469,-10.4699901375332,
0.554282497694829));
#30553=CARTESIAN_POINT('Ctrl Pts',(-6.22832465486985,-9.47045776483884,
-4.49870562403222));
#30554=CARTESIAN_POINT('Ctrl Pts',(-6.16907609212502,-6.18517442841409,
-8.46590455045353));
#30555=CARTESIAN_POINT('Ctrl Pts',(-6.10982752938018,-1.40706268161673,
-10.3898073695953));
#30556=CARTESIAN_POINT('Ctrl Pts',(-6.05057896663535,3.71065196087965,-9.80606876339935));
#30557=CARTESIAN_POINT('Ctrl Pts',(-5.99133040389051,7.93277881804871,-6.85557749509213));
#30558=CARTESIAN_POINT('Ctrl Pts',(-5.93208184114569,10.2402826148908,-2.25045207335339));
#30559=CARTESIAN_POINT('Ctrl Pts',(-5.87283327840083,10.0762336698203,2.89783325926043));
#30560=CARTESIAN_POINT('Ctrl Pts',(-5.81358471565602,7.4802261654632,7.34670940495238));
#30561=CARTESIAN_POINT('Ctrl Pts',(-5.75433615291117,3.07882185862981,10.0224138075675));
#30562=CARTESIAN_POINT('Ctrl Pts',(-5.69508759016634,-2.06567430345103,
10.2791493927931));
#30563=CARTESIAN_POINT('Ctrl Pts',(-5.63583902742151,-6.7116077616892,8.05495150950825));
#30564=CARTESIAN_POINT('Ctrl Pts',(-5.57659046467666,-9.73765501269281,
3.88664346462016));
#30565=CARTESIAN_POINT('Ctrl Pts',(-5.51734190193184,-10.4134616647286,
-1.21972895535173));
#30566=CARTESIAN_POINT('Ctrl Pts',(-5.458093339187,-8.57591778746981,-6.03171258183405));
#30567=CARTESIAN_POINT('Ctrl Pts',(-5.39884477644216,-4.6685254578629,-9.38790672176614));
#30568=CARTESIAN_POINT('Ctrl Pts',(-5.33959621369733,0.365643087792113,
-10.4782740801931));
#30569=CARTESIAN_POINT('Ctrl Pts',(-5.2803476509525,5.31156151280302,-9.03964804973101));
#30570=CARTESIAN_POINT('Ctrl Pts',(-5.22109908820765,8.975503168763,-5.41924952690144));
#30571=CARTESIAN_POINT('Ctrl Pts',(-5.16185052546283,10.4731540785531,-0.490883096248158));
#30572=CARTESIAN_POINT('Ctrl Pts',(-5.10260196271799,9.44304734211565,4.55596087141438));
#30573=CARTESIAN_POINT('Ctrl Pts',(-5.04335339997316,6.13380530950194,8.50319675136485));
#30574=CARTESIAN_POINT('Ctrl Pts',(-4.98410483722832,1.34413310702038,10.3981358309029));
#30575=CARTESIAN_POINT('Ctrl Pts',(-4.92485627448348,-3.76995356633927,
9.78342336173498));
#30576=CARTESIAN_POINT('Ctrl Pts',(-4.86560771173865,-7.97413966134769,
6.80742383201003));
#30577=CARTESIAN_POINT('Ctrl Pts',(-4.80635914899381,-10.2537200120049,
2.1884123200864));
#30578=CARTESIAN_POINT('Ctrl Pts',(-4.74711058624898,-10.0585044255243,
-2.95878544152915));
#30579=CARTESIAN_POINT('Ctrl Pts',(-4.68786202350414,-7.43560933766978,
-7.3918628467291));
#30580=CARTESIAN_POINT('Ctrl Pts',(-4.62861346075931,-3.01808598246791,
-10.0408704587663));
#30581=CARTESIAN_POINT('Ctrl Pts',(-4.56936489801447,2.12787026524513,-10.2664546315455));
#30582=CARTESIAN_POINT('Ctrl Pts',(-4.51011633526964,6.76025244608102,-8.01416929148315));
#30583=CARTESIAN_POINT('Ctrl Pts',(-4.4508677725248,9.7610077375538,-3.82761681921153));
#30584=CARTESIAN_POINT('Ctrl Pts',(-4.39161920977998,10.4058861118699,1.28275359835361));
#30585=CARTESIAN_POINT('Ctrl Pts',(-4.33237064703513,8.53924236135476,6.08352385228661));
#30586=CARTESIAN_POINT('Ctrl Pts',(-4.2731220842903,4.61160198938182,9.41599966327665));
#30587=CARTESIAN_POINT('Ctrl Pts',(-4.21387352154547,-0.429075783032848,
10.4758682952637));
#30588=CARTESIAN_POINT('Ctrl Pts',(-4.15462495880063,-5.3661935788409,9.00732418877565));
#30589=CARTESIAN_POINT('Ctrl Pts',(-4.09537639605579,-9.00814883351634,
5.36480914483585));
#30590=CARTESIAN_POINT('Ctrl Pts',(-4.03612783331096,-10.4759341178572,
0.427465701094278));
#30591=CARTESIAN_POINT('Ctrl Pts',(-3.97687927056613,-9.41529077705088,
-4.61304911646044));
#30592=CARTESIAN_POINT('Ctrl Pts',(-3.91763070782129,-6.08221135112264,
-8.54017726089867));
#30593=CARTESIAN_POINT('Ctrl Pts',(-3.85838214507646,-1.28115426216585,
-10.4060831403478));
#30594=CARTESIAN_POINT('Ctrl Pts',(-3.79913358233163,3.8291169811801,-9.76041934097784));
#30595=CARTESIAN_POINT('Ctrl Pts',(-3.73988501958678,8.01520820627361,-6.75902063744299));
#30596=CARTESIAN_POINT('Ctrl Pts',(-3.68063645684196,10.2667815509319,-2.12629234884133));
#30597=CARTESIAN_POINT('Ctrl Pts',(-3.62138789409711,10.0404064788223,3.01962916718597));
#30598=CARTESIAN_POINT('Ctrl Pts',(-3.56213933135229,7.39071995175672,7.43674533394825));
#30599=CARTESIAN_POINT('Ctrl Pts',(-3.50289076860744,2.95723947598601,10.0589590539462));
#30600=CARTESIAN_POINT('Ctrl Pts',(-3.44364220586262,-2.18998822827795,
10.2533835453132));
#30601=CARTESIAN_POINT('Ctrl Pts',(-3.38439364311777,-6.80864932809227,
7.97309330776734));
#30602=CARTESIAN_POINT('Ctrl Pts',(-3.32514508037295,-9.78400266498433,
3.76844986949217));
#30603=CARTESIAN_POINT('Ctrl Pts',(-3.26589651762811,-10.3979291230557,
-1.34573122101146));
#30604=CARTESIAN_POINT('Ctrl Pts',(-3.20664795488328,-8.50225392258195,
-6.13511212637845));
#30605=CARTESIAN_POINT('Ctrl Pts',(-3.14739939213844,-4.55450947899581,
-9.44374745389952));
#30606=CARTESIAN_POINT('Ctrl Pts',(-3.08815082939361,0.492492750162627,
-10.4730785091268));
#30607=CARTESIAN_POINT('Ctrl Pts',(-3.02890226664877,5.42062894282451,-8.97467015725421));
#30608=CARTESIAN_POINT('Ctrl Pts',(-2.96965370390394,9.04046429747557,-5.31017211146357));
#30609=CARTESIAN_POINT('Ctrl Pts',(-2.9104051411591,10.478330153541,-0.36403263684834));
#30610=CARTESIAN_POINT('Ctrl Pts',(-2.85115657841426,9.38718908708332,4.66996826655597));
#30611=CARTESIAN_POINT('Ctrl Pts',(-2.79190801566943,6.03039444449335,8.57684472350524));
#30612=CARTESIAN_POINT('Ctrl Pts',(-2.7326594529246,1.21812845559219,10.4136490066149));
#30613=CARTESIAN_POINT('Ctrl Pts',(-2.67341089017976,-3.88814003672063,
9.73705754435836));
#30614=CARTESIAN_POINT('Ctrl Pts',(-2.61416232743493,-8.05598294742662,
6.71036968564828));
#30615=CARTESIAN_POINT('Ctrl Pts',(-2.55491376469009,-10.2794667528907,
2.06409443667468));
#30616=CARTESIAN_POINT('Ctrl Pts',(-2.49566520194525,-10.0219404931087,
-3.08036220595614));
#30617=CARTESIAN_POINT('Ctrl Pts',(-2.43641663920042,-7.34555965317983,
-7.48135522140693));
#30618=CARTESIAN_POINT('Ctrl Pts',(-2.37716807645559,-2.8962845695608,-10.0766789300553));
#30619=CARTESIAN_POINT('Ctrl Pts',(-2.31791951371075,2.25202591556642,-10.2399366132273));
#30620=CARTESIAN_POINT('Ctrl Pts',(-2.25867095096592,6.85679663369709,-7.93172506403346));
#30621=CARTESIAN_POINT('Ctrl Pts',(-2.19942238822108,9.80663895208724,-3.70914478427321));
#30622=CARTESIAN_POINT('Ctrl Pts',(-2.14017382547625,10.3895909899559,1.40865951483102));
#30623=CARTESIAN_POINT('Ctrl Pts',(-2.08092526273141,8.46495382699166,6.18647551310075));
#30624=CARTESIAN_POINT('Ctrl Pts',(-2.02167669998658,4.49725001947583,9.47114907651764));
#30625=CARTESIAN_POINT('Ctrl Pts',(-1.96242813724174,-0.555891664582547,
10.4699048240442));
#30626=CARTESIAN_POINT('Ctrl Pts',(-1.90317957449691,-5.47486560938269,
8.941687152126));
#30627=CARTESIAN_POINT('Ctrl Pts',(-1.84393101175207,-9.072448376092,5.25534042954797));
#30628=CARTESIAN_POINT('Ctrl Pts',(-1.78468244900724,-10.4803420977758,
0.300586228699219));
#30629=CARTESIAN_POINT('Ctrl Pts',(-1.7254338862624,-9.35874330230254,-4.72671623528466));
#30630=CARTESIAN_POINT('Ctrl Pts',(-1.66618532351757,-5.97835648900369,
-8.61319779510975));
#30631=CARTESIAN_POINT('Ctrl Pts',(-1.60693676077273,-1.15505799756011,
-10.4208331523717));
#30632=CARTESIAN_POINT('Ctrl Pts',(-1.5476881980279,3.94702056942422,-9.71333882822164));
#30633=CARTESIAN_POINT('Ctrl Pts',(-1.48843963528306,8.0964623901765,-6.66147275996483));
#30634=CARTESIAN_POINT('Ctrl Pts',(-1.42919107253823,10.2917751528953,-2.00182086349988));
#30635=CARTESIAN_POINT('Ctrl Pts',(-1.36994250979339,10.0031071452691,3.14098233162225));
#30636=CARTESIAN_POINT('Ctrl Pts',(-1.31069394704856,7.30013009732543,7.52569087389453));
#30637=CARTESIAN_POINT('Ctrl Pts',(-1.25144538430372,2.83522349754239,10.0940294375576));
#30638=CARTESIAN_POINT('Ctrl Pts',(-1.19219682155889,-2.31398105307032,
10.2261143281957));
#30639=CARTESIAN_POINT('Ctrl Pts',(-1.13294825881405,-6.90469259801799,
7.89006607666695));
#30640=CARTESIAN_POINT('Ctrl Pts',(-1.07369969606922,-9.82891576911162,
3.64970373742945));
#30641=CARTESIAN_POINT('Ctrl Pts',(-1.01445113332438,-10.380872018211,-1.47153617312628));
#30642=CARTESIAN_POINT('Ctrl Pts',(-0.955202570579548,-8.42734344184841,
-6.23761212968768));
#30643=CARTESIAN_POINT('Ctrl Pts',(-0.895954007834717,-4.43982570971225,
-9.49820352670374));
#30644=CARTESIAN_POINT('Ctrl Pts',(-0.836705445089881,0.619270202354978,
-10.4663473563483));
#30645=CARTESIAN_POINT('Ctrl Pts',(-0.777456882345046,5.52890159042847,
-8.90837638241207));
#30646=CARTESIAN_POINT('Ctrl Pts',(-0.71820831960021,9.10409989696232,-5.20031610898184));
#30647=CARTESIAN_POINT('Ctrl Pts',(-0.658959756855376,10.4819698768157,
-0.237128802336295));
#30648=CARTESIAN_POINT('Ctrl Pts',(-0.599711194110542,9.32995446540496,
4.78329094252682));
#30649=CARTESIAN_POINT('Ctrl Pts',(-0.540462631365705,5.92609939215782,
8.64923514311966));
#30650=CARTESIAN_POINT('Ctrl Pts',(-0.481214068620872,1.09194519994383,
10.4276353143587));
#30651=CARTESIAN_POINT('Ctrl Pts',(-0.421965505876034,-4.0057564209339,
9.68926406183886));
#30652=CARTESIAN_POINT('Ctrl Pts',(-0.362716943131203,-8.13664505080342,
6.61233165305132));
#30653=CARTESIAN_POINT('Ctrl Pts',(-0.303468380386365,-10.3037062996053,
1.93947391141822));
#30654=CARTESIAN_POINT('Ctrl Pts',(-0.244219817641532,-9.98390712597543,
-3.20148732097496));
#30655=CARTESIAN_POINT('Ctrl Pts',(-0.184971254896697,-7.25443294882962,
-7.56975066843671));
#30656=CARTESIAN_POINT('Ctrl Pts',(-0.125722692151862,-2.7740584993699,
-10.1110099362393));
#30657=CARTESIAN_POINT('Ctrl Pts',(-0.0664741294070278,2.37585137208773,
-10.211917205029));
#30658=CARTESIAN_POINT('Ctrl Pts',(-0.00722556666219231,6.95233546092519,
-7.848117856984));
#30659=CARTESIAN_POINT('Ctrl Pts',(0.0520229960826416,9.85083230810637,
-3.59012893818949));
#30660=CARTESIAN_POINT('Ctrl Pts',(0.111271558827477,10.3717725107696,1.53435894975116));
#30661=CARTESIAN_POINT('Ctrl Pts',(0.170520121572311,8.38942417794793,6.28851998843207));
#30662=CARTESIAN_POINT('Ctrl Pts',(0.229768684317148,4.38223859253949,9.52491003146027));
#30663=CARTESIAN_POINT('Ctrl Pts',(0.289017247061982,-0.682625920371043,
10.4624058141013));
#30664=CARTESIAN_POINT('Ctrl Pts',(0.348265809806817,-5.58273513680522,
8.8747398847227));
#30665=CARTESIAN_POINT('Ctrl Pts',(0.407514372551651,-9.13541725268214,
5.14509959176606));
#30666=CARTESIAN_POINT('Ctrl Pts',(0.466762935296485,-10.4832142945652,
0.173665725238765));
#30667=CARTESIAN_POINT('Ctrl Pts',(0.52601149804132,-9.30082196402671,-4.8396961877274));
#30668=CARTESIAN_POINT('Ctrl Pts',(0.585260060786157,-5.87362828986304,
-8.68494410471449));
#30669=CARTESIAN_POINT('Ctrl Pts',(0.644508623530991,-1.02878615726,-10.4340771460299));
#30670=CARTESIAN_POINT('Ctrl Pts',(0.703757186275826,4.0643334282463,-9.66479182544668));
#30671=CARTESIAN_POINT('Ctrl Pts',(0.763005749020661,8.1765526549945,-6.56302991227287));
#30672=CARTESIAN_POINT('Ctrl Pts',(0.822254311765496,10.3152148975558,-1.8768974633799));
#30673=CARTESIAN_POINT('Ctrl Pts',(0.88150287451033,9.96442833619652,3.26156383705692));
#30674=CARTESIAN_POINT('Ctrl Pts',(0.940751437255166,7.20829597612923,7.61418408655239));
#30675=CARTESIAN_POINT('Ctrl Pts',(0.980250479085055,4.21155540437341,9.28866001522528));
#30676=CARTESIAN_POINT('Ctrl Pts',(1.,2.60344811511698,9.71940883564396));
#30677=CARTESIAN_POINT('Ctrl Pts',(1.,2.60344811511698,9.71940883564396));
#30678=CARTESIAN_POINT('Ctrl Pts',(1.,2.84069167774707,9.6506072019626));
#30679=CARTESIAN_POINT('Ctrl Pts',(1.00000000000001,3.07490714309636,9.57303457599562));
#30680=CARTESIAN_POINT('Ctrl Pts',(1.,3.30569472464045,9.48703944558796));
#30681=CARTESIAN_POINT('Ctrl Pts',(1.,3.53907106298549,9.40007970314528));
#30682=CARTESIAN_POINT('Ctrl Pts',(1.,3.76894275222114,9.30450718872403));
#30683=CARTESIAN_POINT('Ctrl Pts',(1.,3.99488366234361,9.2006301234426));
#30684=CARTESIAN_POINT('Ctrl Pts',(1.,4.22183130088218,9.09629021151094));
#30685=CARTESIAN_POINT('Ctrl Pts',(1.,4.44481362873405,8.98357126478796));
#30686=CARTESIAN_POINT('Ctrl Pts',(1.,4.66337739592737,8.86273774043803));
#30687=CARTESIAN_POINT('Ctrl Pts',(1.,4.88031644999598,8.74280244279529));
#30688=CARTESIAN_POINT('Ctrl Pts',(0.999999999999998,5.09290290626542,8.61487237722491));
#30689=CARTESIAN_POINT('Ctrl Pts',(0.999999999999998,5.30066443456372,8.47916440146929));
#30690=CARTESIAN_POINT('Ctrl Pts',(0.999999999999998,5.43935724551385,8.38857149536169));
#30691=CARTESIAN_POINT('Ctrl Pts',(0.999999999999999,5.57589930057551,8.29451164480296));
#30692=CARTESIAN_POINT('Ctrl Pts',(0.999999999999998,5.71014105120108,8.19704013131701));
#30693=CARTESIAN_POINT('Ctrl Pts',(0.999999999999998,5.81242655791967,8.12277170810978));
#30694=CARTESIAN_POINT('Ctrl Pts',(1.,5.9133764403282,8.04652243031488));
#30695=CARTESIAN_POINT('Ctrl Pts',(1.,6.01292125894988,7.96831413748024));
#30696=CARTESIAN_POINT('Ctrl Pts',(1.,6.03974575183923,7.94723923047776));
#30697=CARTESIAN_POINT('Ctrl Pts',(1.,6.06647063088991,7.92602003751734));
#30698=CARTESIAN_POINT('Ctrl Pts',(1.,6.09307495250317,7.90467285051554));
#30699=CARTESIAN_POINT('Ctrl Pts',(1.,6.28715174484022,7.74894651255607));
#30700=CARTESIAN_POINT('Ctrl Pts',(0.999999999999995,6.47502692283882,7.58624843803383));
#30701=CARTESIAN_POINT('Ctrl Pts',(0.999999999999996,6.65627725204656,7.41686189931922));
#30702=CARTESIAN_POINT('Ctrl Pts',(0.999999999999996,6.72100528412185,7.35637065850897));
#30703=CARTESIAN_POINT('Ctrl Pts',(0.999999999999999,6.78488816611234,7.29502599747633));
#30704=CARTESIAN_POINT('Ctrl Pts',(0.999999999999999,6.84790570190959,7.23283949466907));
#30705=CARTESIAN_POINT('Ctrl Pts',(1.,7.02385871161102,7.05920683523047));
#30706=CARTESIAN_POINT('Ctrl Pts',(1.,7.19306826910953,6.87901391023897));
#30707=CARTESIAN_POINT('Ctrl Pts',(1.,7.35530118582863,6.69274096896221));
#30708=CARTESIAN_POINT('Ctrl Pts',(1.,7.51824283801115,6.50565427026784));
#30709=CARTESIAN_POINT('Ctrl Pts',(1.,7.67414712093029,6.31243376066224));
#30710=CARTESIAN_POINT('Ctrl Pts',(1.,7.82273682237407,6.1135329641478));
#30711=CARTESIAN_POINT('Ctrl Pts',(1.,7.97083959347484,5.91528396807531));
#30712=CARTESIAN_POINT('Ctrl Pts',(1.,8.11167595875326,5.71139127016028));
#30713=CARTESIAN_POINT('Ctrl Pts',(1.,8.24492584265527,5.50227978289586));
#30714=CARTESIAN_POINT('Ctrl Pts',(1.,8.30521405441425,5.40766838620072));
#30715=CARTESIAN_POINT('Ctrl Pts',(0.999999999999997,8.36394861758055,5.3119883953279));
#30716=CARTESIAN_POINT('Ctrl Pts',(0.999999999999997,8.42109653790941,5.21527801938325));
#30717=CARTESIAN_POINT('Ctrl Pts',(0.999999999999997,8.45087438326695,5.16488551861022));
#30718=CARTESIAN_POINT('Ctrl Pts',(0.999999999999998,8.48022140378265,5.11421324826767));
#30719=CARTESIAN_POINT('Ctrl Pts',(0.999999999999998,8.50913269400644,5.06326655825364));
#30720=CARTESIAN_POINT('Ctrl Pts',(0.999999999999998,8.52853358179415,5.0290788409824));
#30721=CARTESIAN_POINT('Ctrl Pts',(0.999999999999996,8.54774115151347,4.99476217267899));
#30722=CARTESIAN_POINT('Ctrl Pts',(0.999999999999996,8.56673757646602,4.96034807967986));
#30723=CARTESIAN_POINT('Ctrl Pts',(0.999999999999996,8.68625359767795,4.74383178889639));
#30724=CARTESIAN_POINT('Ctrl Pts',(1.,8.79751973028822,4.52328346537184));
#30725=CARTESIAN_POINT('Ctrl Pts',(1.,8.90031168588408,4.29917497997117));
#30726=CARTESIAN_POINT('Ctrl Pts',(1.,9.00301015821637,4.07527030811298));
#30727=CARTESIAN_POINT('Ctrl Pts',(0.999999999999998,9.09725016618283,3.84781136171468));
#30728=CARTESIAN_POINT('Ctrl Pts',(0.999999999999998,9.18276364450296,3.61724215327469));
#30729=CARTESIAN_POINT('Ctrl Pts',(0.999999999999999,9.25013088715846,3.43560047386934));
#30730=CARTESIAN_POINT('Ctrl Pts',(0.999999999999997,9.31208142209733,3.25202787668663));
#30731=CARTESIAN_POINT('Ctrl Pts',(0.999999999999997,9.36846285698885,3.06673337277954));
#30732=CARTESIAN_POINT('Ctrl Pts',(0.999999999999998,9.44021348938853,2.83092884135711));
#30733=CARTESIAN_POINT('Ctrl Pts',(0.999999999999998,9.50294665239736,2.59233553672004));
#30734=CARTESIAN_POINT('Ctrl Pts',(0.999999999999998,9.55662998734371,2.35147826686192));
#30735=CARTESIAN_POINT('Ctrl Pts',(0.999999999999999,9.5940332087379,2.18366384553536));
#30736=CARTESIAN_POINT('Ctrl Pts',(0.999999999999998,9.62704217123799,2.01475016264279));
#30737=CARTESIAN_POINT('Ctrl Pts',(0.999999999999998,9.6556309798987,1.84491423498701));
#30738=CARTESIAN_POINT('Ctrl Pts',(0.999999999999998,9.66985502089958,1.76041427463296));
#30739=CARTESIAN_POINT('Ctrl Pts',(1.,9.68298468440151,1.67568602475725));
#30740=CARTESIAN_POINT('Ctrl Pts',(1.,9.69501564091497,1.59075139934658));
#30741=CARTESIAN_POINT('Ctrl Pts',(1.,9.70329996440281,1.53226677998714));
#30742=CARTESIAN_POINT('Ctrl Pts',(0.999999999999997,9.71106332257942,1.47368430996418));
#30743=CARTESIAN_POINT('Ctrl Pts',(0.999999999999997,9.71830409201168,1.41501118134328));
#30744=CARTESIAN_POINT('Ctrl Pts',(0.999999999999997,9.7217772471656,1.38686764204501));
#30745=CARTESIAN_POINT('Ctrl Pts',(1.,9.72513022957085,1.35870230879726));
#30746=CARTESIAN_POINT('Ctrl Pts',(1.,9.7283610524273,1.33053267129302));
#30747=CARTESIAN_POINT('Ctrl Pts',(1.,9.75621798311309,1.08764729061324));
#30748=CARTESIAN_POINT('Ctrl Pts',(0.999999999999999,9.77503411297353,0.844154061252829));
#30749=CARTESIAN_POINT('Ctrl Pts',(0.999999999999999,9.78485426406749,0.600570610607425));
#30750=CARTESIAN_POINT('Ctrl Pts',(0.999999999999999,9.79474459297459,0.355246437877215));
#30751=CARTESIAN_POINT('Ctrl Pts',(0.999999999999998,9.79550996768915,0.109830095075824));
#30752=CARTESIAN_POINT('Ctrl Pts',(0.999999999999997,9.78714427532281,-0.135157539340118));
#30753=CARTESIAN_POINT('Ctrl Pts',(0.999999999999997,9.77880542326125,-0.379359160777594));
#30754=CARTESIAN_POINT('Ctrl Pts',(0.999999999999999,9.76139398474161,-0.623135475248794));
#30755=CARTESIAN_POINT('Ctrl Pts',(0.999999999999998,9.73485233230931,-0.865968606386387));
#30756=CARTESIAN_POINT('Ctrl Pts',(0.999999999999998,9.70865279306758,-1.10567169814608));
#30757=CARTESIAN_POINT('Ctrl Pts',(0.999999999999997,9.67355680745553,-1.3444563628419));
#30758=CARTESIAN_POINT('Ctrl Pts',(0.999999999999997,9.62945950993569,-1.58181327268759));
#30759=CARTESIAN_POINT('Ctrl Pts',(0.999999999999997,9.6192529840039,-1.63675064054647));
#30760=CARTESIAN_POINT('Ctrl Pts',(0.999999999999998,9.60856403800696,-1.69161145235431));
#30761=CARTESIAN_POINT('Ctrl Pts',(0.999999999999998,9.59739099453272,-1.74638925350567));
#30762=CARTESIAN_POINT('Ctrl Pts',(0.999999999999999,9.55734323773339,-1.94273039041888));
#30763=CARTESIAN_POINT('Ctrl Pts',(0.999999999999998,9.51107764815899,-2.13800595497268));
#30764=CARTESIAN_POINT('Ctrl Pts',(0.999999999999998,9.45868910149449,-2.33194450538573));
#30765=CARTESIAN_POINT('Ctrl Pts',(0.999999999999998,9.44806060011906,-2.37129043653008));
#30766=CARTESIAN_POINT('Ctrl Pts',(0.999999999999997,9.43717863629369,-2.41058591625719));
#30767=CARTESIAN_POINT('Ctrl Pts',(0.999999999999997,9.42605224796243,-2.44979991766584));
#30768=CARTESIAN_POINT('Ctrl Pts',(0.999999999999997,9.35956117629125,-2.68414199710326));
#30769=CARTESIAN_POINT('Ctrl Pts',(0.999999999999997,9.28429949892928,-2.91575317404239));
#30770=CARTESIAN_POINT('Ctrl Pts',(0.999999999999997,9.2005384559038,-3.14417935336596));
#30771=CARTESIAN_POINT('Ctrl Pts',(0.999999999999997,9.11644482312329,-3.3735125439239));
#30772=CARTESIAN_POINT('Ctrl Pts',(0.999999999999997,9.02378391757509,-3.59963600047152));
#30773=CARTESIAN_POINT('Ctrl Pts',(0.999999999999997,8.92278109951216,-3.82207197411459));
#30774=CARTESIAN_POINT('Ctrl Pts',(0.999999999999997,8.83217822944176,-4.02160440306533));
#30775=CARTESIAN_POINT('Ctrl Pts',(0.999999999999999,8.73486209429878,-4.21816969086207));
#30776=CARTESIAN_POINT('Ctrl Pts',(0.999999999999998,8.6309646900063,-4.41140453007061));
#30777=CARTESIAN_POINT('Ctrl Pts',(0.999999999999998,8.6132277511296,-4.4443927895486));
#30778=CARTESIAN_POINT('Ctrl Pts',(0.999999999999999,8.59529894366689,-4.47728393785859));
#30779=CARTESIAN_POINT('Ctrl Pts',(0.999999999999999,8.57717884575786,-4.51007610455165));
#30780=CARTESIAN_POINT('Ctrl Pts',(0.999999999999999,8.56101090653111,-4.5393354253825));
#30781=CARTESIAN_POINT('Ctrl Pts',(0.999999999999998,8.54469196169516,-4.56851353632572));
#30782=CARTESIAN_POINT('Ctrl Pts',(0.999999999999998,8.52822781333363,-4.59759993645712));
#30783=CARTESIAN_POINT('Ctrl Pts',(0.999999999999998,8.40828069815436,-4.80950459803457));
#30784=CARTESIAN_POINT('Ctrl Pts',(0.999999999999999,8.28055247410411,-5.01668529771194));
#30785=CARTESIAN_POINT('Ctrl Pts',(0.999999999999999,8.14527406560948,-5.21867494622436));
#30786=CARTESIAN_POINT('Ctrl Pts',(0.999999999999999,8.01107412784125,-5.41905428659241));
#30787=CARTESIAN_POINT('Ctrl Pts',(1.,7.86944355538485,-5.61432554891969));
#30788=CARTESIAN_POINT('Ctrl Pts',(1.,7.72056576365074,-5.80400382354972));
#30789=CARTESIAN_POINT('Ctrl Pts',(1.,7.65750044054917,-5.88435242044626));
#30790=CARTESIAN_POINT('Ctrl Pts',(1.,7.59313418212457,-5.96369700362708));
#30791=CARTESIAN_POINT('Ctrl Pts',(1.,7.52747886047206,-6.04199877428964));
#30792=CARTESIAN_POINT('Ctrl Pts',(1.,7.42746573325124,-6.1612763096635));
#30793=CARTESIAN_POINT('Ctrl Pts',(1.,7.32446160350885,-6.27813437307676));
#30794=CARTESIAN_POINT('Ctrl Pts',(1.,7.21857426272793,-6.39248696093098));
#30795=CARTESIAN_POINT('Ctrl Pts',(-8.,7.21801009705396,-6.39216838336781));
#30796=CARTESIAN_POINT('Ctrl Pts',(-8.,7.380337662993,-6.21660080725665));
#30797=CARTESIAN_POINT('Ctrl Pts',(-8.,7.53570853367131,-6.03520943062631));
#30798=CARTESIAN_POINT('Ctrl Pts',(-8.,7.68398049959171,-5.84850779751532));
#30799=CARTESIAN_POINT('Ctrl Pts',(-8.,7.83425278465447,-5.65928739527419));
#30800=CARTESIAN_POINT('Ctrl Pts',(-8.,7.97723370551244,-5.46461203049959));
#30801=CARTESIAN_POINT('Ctrl Pts',(-8.,8.1127416114141,-5.26497403764809));
#30802=CARTESIAN_POINT('Ctrl Pts',(-8.,8.24926768438102,-5.06383602287576));
#30803=CARTESIAN_POINT('Ctrl Pts',(-8.,8.37820838989442,-4.85765999894323));
#30804=CARTESIAN_POINT('Ctrl Pts',(-8.,8.49933848010934,-4.64691438626471));
#30805=CARTESIAN_POINT('Ctrl Pts',(-8.,8.6201424258609,-4.43673620909814));
#30806=CARTESIAN_POINT('Ctrl Pts',(-8.,8.733178071977,-4.22201244059188));
#30807=CARTESIAN_POINT('Ctrl Pts',(-8.,8.83817785999191,-4.00318131294289));
#30808=CARTESIAN_POINT('Ctrl Pts',(-8.,8.90711924309347,-3.85949987423702));
#30809=CARTESIAN_POINT('Ctrl Pts',(-8.,8.97259541777826,-3.71404720995258));
#30810=CARTESIAN_POINT('Ctrl Pts',(-8.,9.03451925692504,-3.56694295599801));
#30811=CARTESIAN_POINT('Ctrl Pts',(-8.,9.0602105812632,-3.50591148327374));
#30812=CARTESIAN_POINT('Ctrl Pts',(-8.,9.08529032912163,-3.44459568829976));
#30813=CARTESIAN_POINT('Ctrl Pts',(-8.,9.10975179059862,-3.38300398939247));
#30814=CARTESIAN_POINT('Ctrl Pts',(-8.,9.12543389087233,-3.34351791047601));
#30815=CARTESIAN_POINT('Ctrl Pts',(-8.,9.1408618685122,-3.30391843322633));
#30816=CARTESIAN_POINT('Ctrl Pts',(-8.,9.15603389139516,-3.26420776351618));
#30817=CARTESIAN_POINT('Ctrl Pts',(-8.,9.16539707181774,-3.23970093485752));
#30818=CARTESIAN_POINT('Ctrl Pts',(-8.,9.17466357769889,-3.21514958524345));
#30819=CARTESIAN_POINT('Ctrl Pts',(-8.,9.18383032373706,-3.19056134096833));
#30820=CARTESIAN_POINT('Ctrl Pts',(-8.,9.26956766576029,-2.96058543671737));
#30821=CARTESIAN_POINT('Ctrl Pts',(-8.,9.34642836267942,-2.72780037578161));
#30822=CARTESIAN_POINT('Ctrl Pts',(-8.,9.41421809880825,-2.49269184582416));
#30823=CARTESIAN_POINT('Ctrl Pts',(-8.,9.44158158155583,-2.39778974750246));
#30824=CARTESIAN_POINT('Ctrl Pts',(-8.,9.46746660052344,-2.30250872996448));
#30825=CARTESIAN_POINT('Ctrl Pts',(-8.,9.49185833340935,-2.20687947232321));
#30826=CARTESIAN_POINT('Ctrl Pts',(-8.,9.55185317751319,-1.97166607314452));
#30827=CARTESIAN_POINT('Ctrl Pts',(-8.,9.60281745079054,-1.73434714094384));
#30828=CARTESIAN_POINT('Ctrl Pts',(-8.,9.64482582839825,-1.49544885170401));
#30829=CARTESIAN_POINT('Ctrl Pts',(-8.,9.687149082017,-1.25475988773113));
#30830=CARTESIAN_POINT('Ctrl Pts',(-8.,9.72038175363905,-1.01246716488642));
#30831=CARTESIAN_POINT('Ctrl Pts',(-8.,9.74454885870802,-0.769095294744196));
#30832=CARTESIAN_POINT('Ctrl Pts',(-8.,9.76872028978328,-0.525679860085804));
#30833=CARTESIAN_POINT('Ctrl Pts',(-8.,9.78382293411453,-0.281184228473798));
#30834=CARTESIAN_POINT('Ctrl Pts',(-8.,9.78982997440973,-0.0361296562227952));
#30835=CARTESIAN_POINT('Ctrl Pts',(-8.,9.79255533923483,0.0750504056083886));
#30836=CARTESIAN_POINT('Ctrl Pts',(-8.,9.79340776314294,0.186345508045464));
#30837=CARTESIAN_POINT('Ctrl Pts',(-8.,9.79238119762556,0.297706651553354));
#30838=CARTESIAN_POINT('Ctrl Pts',(-8.,9.79184842307034,0.355501680410697));
#30839=CARTESIAN_POINT('Ctrl Pts',(-8.,9.79080951024432,0.413314491676565));
#30840=CARTESIAN_POINT('Ctrl Pts',(-8.,9.78926337738701,0.471138189497998));
#30841=CARTESIAN_POINT('Ctrl Pts',(-8.,9.78827687496122,0.50803231402231));
#30842=CARTESIAN_POINT('Ctrl Pts',(-8.,9.78708363293494,0.544935840717242));
#30843=CARTESIAN_POINT('Ctrl Pts',(-8.,9.78568466161457,0.581816587647619));
#30844=CARTESIAN_POINT('Ctrl Pts',(-8.,9.77634732562296,0.827974547211403));
#30845=CARTESIAN_POINT('Ctrl Pts',(-8.,9.75784567918533,1.07334629644098));
#30846=CARTESIAN_POINT('Ctrl Pts',(-8.,9.73025873568655,1.31740270617224));
#30847=CARTESIAN_POINT('Ctrl Pts',(-8.,9.70256576677612,1.56239710242996));
#30848=CARTESIAN_POINT('Ctrl Pts',(-8.,9.66571755991781,1.80606669459938));
#30849=CARTESIAN_POINT('Ctrl Pts',(-8.,9.61974208798732,2.04788261285709));
#30850=CARTESIAN_POINT('Ctrl Pts',(-8.,9.58407745535832,2.2354668947878));
#30851=CARTESIAN_POINT('Ctrl Pts',(-8.,9.54291936511459,2.42193593333913));
#30852=CARTESIAN_POINT('Ctrl Pts',(-8.,9.49625929589928,2.60704160924379));
#30853=CARTESIAN_POINT('Ctrl Pts',(-8.,9.43617821052004,2.84538994659596));
#30854=CARTESIAN_POINT('Ctrl Pts',(-8.,9.36697643674185,3.08147866016247));
#30855=CARTESIAN_POINT('Ctrl Pts',(-8.,9.28891878956949,3.31486179503419));
#30856=CARTESIAN_POINT('Ctrl Pts',(-8.,9.23376423793927,3.47976738248396));
#30857=CARTESIAN_POINT('Ctrl Pts',(-8.,9.17418715731129,3.64332194306396));
#30858=CARTESIAN_POINT('Ctrl Pts',(-8.,9.11026643845191,3.8053622791706));
#30859=CARTESIAN_POINT('Ctrl Pts',(-8.,9.07823135006152,3.88657188667525));
#30860=CARTESIAN_POINT('Ctrl Pts',(-8.,9.04510508571049,3.96740107672111));
#30861=CARTESIAN_POINT('Ctrl Pts',(-8.,9.01089650850777,4.04782870220661));
#30862=CARTESIAN_POINT('Ctrl Pts',(-8.,8.98491018599784,4.10892502323126));
#30863=CARTESIAN_POINT('Ctrl Pts',(-8.,8.95829929144517,4.16978960999898));
#30864=CARTESIAN_POINT('Ctrl Pts',(-8.,8.93106744624091,4.2304130132153));
#30865=CARTESIAN_POINT('Ctrl Pts',(-8.,8.91985556199095,4.25537285617128));
#30866=CARTESIAN_POINT('Ctrl Pts',(-8.,8.90854177922313,4.2802842982631));
#30867=CARTESIAN_POINT('Ctrl Pts',(-8.,8.89712828878493,4.30514299630826));
#30868=CARTESIAN_POINT('Ctrl Pts',(-8.,8.79449435935336,4.52868073655892));
#30869=CARTESIAN_POINT('Ctrl Pts',(-8.,8.68375805043763,4.74805239503432));
#30870=CARTESIAN_POINT('Ctrl Pts',(-8.,8.56525012527811,4.96284306665098));
#30871=CARTESIAN_POINT('Ctrl Pts',(-8.,8.44538164369718,5.18009969003529));
#30872=CARTESIAN_POINT('Ctrl Pts',(-8.,8.31756185464637,5.39267013945067));
#30873=CARTESIAN_POINT('Ctrl Pts',(-8.,8.18208202554571,5.60011073616086));
#30874=CARTESIAN_POINT('Ctrl Pts',(-8.,8.04666337133259,5.80745766464561));
#30875=CARTESIAN_POINT('Ctrl Pts',(-8.,7.9035912805775,6.00967995783845));
#30876=CARTESIAN_POINT('Ctrl Pts',(-8.,7.75311010158105,6.20631140538698));
#30877=CARTESIAN_POINT('Ctrl Pts',(-8.,7.60409269401218,6.40103016527181));
#30878=CARTESIAN_POINT('Ctrl Pts',(-8.,7.44780928129002,6.59026684301417));
#30879=CARTESIAN_POINT('Ctrl Pts',(-8.,7.2844565981824,6.77353780787826));
#30880=CARTESIAN_POINT('Ctrl Pts',(-8.,7.25089455072778,6.8111922173609));
#30881=CARTESIAN_POINT('Ctrl Pts',(-8.,7.21703396184226,6.84859467696372));
#30882=CARTESIAN_POINT('Ctrl Pts',(-8.,7.18287634384795,6.88574079722686));
#30883=CARTESIAN_POINT('Ctrl Pts',(-8.,7.04310058845776,7.03774574735134));
#30884=CARTESIAN_POINT('Ctrl Pts',(-8.,6.89835220047973,7.18545984496082));
#30885=CARTESIAN_POINT('Ctrl Pts',(-8.,6.748868793449,7.32870634277334));
#30886=CARTESIAN_POINT('Ctrl Pts',(-8.,6.72044536021718,7.35594386262349));
#30887=CARTESIAN_POINT('Ctrl Pts',(-8.,6.6918476905919,7.38302252032495));
#30888=CARTESIAN_POINT('Ctrl Pts',(-8.,6.66309763711236,7.40992229604933));
#30889=CARTESIAN_POINT('Ctrl Pts',(-8.,6.48228035952991,7.57910264966232));
#30890=CARTESIAN_POINT('Ctrl Pts',(-8.,6.29529505695125,7.74135050059987));
#30891=CARTESIAN_POINT('Ctrl Pts',(-8.,6.10262671834098,7.89643860443478));
#30892=CARTESIAN_POINT('Ctrl Pts',(-8.,5.90856001007317,8.0526523239272));
#30893=CARTESIAN_POINT('Ctrl Pts',(-8.,5.70872697509029,8.20160239784391));
#30894=CARTESIAN_POINT('Ctrl Pts',(-8.,5.50358539266632,8.34301978271322));
#30895=CARTESIAN_POINT('Ctrl Pts',(-8.,5.31584799310374,8.47243933663592));
#30896=CARTESIAN_POINT('Ctrl Pts',(-8.,5.12366384911883,8.5955499246735));
#30897=CARTESIAN_POINT('Ctrl Pts',(-8.,4.92736179531277,8.71211422557509));
#30898=CARTESIAN_POINT('Ctrl Pts',(-8.,4.89295954023047,8.73254230941505));
#30899=CARTESIAN_POINT('Ctrl Pts',(-8.,4.85843076693046,8.75276925692888));
#30900=CARTESIAN_POINT('Ctrl Pts',(-8.,4.82377719165751,8.77279368760958));
#30901=CARTESIAN_POINT('Ctrl Pts',(-8.,4.79450813280393,8.78970669688745));
#30902=CARTESIAN_POINT('Ctrl Pts',(-8.,4.76515157202874,8.80647430503471));
#30903=CARTESIAN_POINT('Ctrl Pts',(-8.,4.73571877014772,8.82309008094362));
#30904=CARTESIAN_POINT('Ctrl Pts',(-8.,4.5175174124504,8.94627185878366));
#30905=CARTESIAN_POINT('Ctrl Pts',(-8.,4.29497552947991,9.0612009825643));
#30906=CARTESIAN_POINT('Ctrl Pts',(-8.,4.06855852697811,9.16761501762388));
#30907=CARTESIAN_POINT('Ctrl Pts',(-8.,3.84298108906434,9.27363446458045));
#30908=CARTESIAN_POINT('Ctrl Pts',(-8.,3.61355665285897,9.37120219380835));
#30909=CARTESIAN_POINT('Ctrl Pts',(-8.,3.38071837058219,9.46001495319009));
#30910=CARTESIAN_POINT('Ctrl Pts',(-8.,3.27719791908491,9.49950131625726));
#30911=CARTESIAN_POINT('Ctrl Pts',(-8.,3.17300234029469,9.53725646338326));
#30912=CARTESIAN_POINT('Ctrl Pts',(-8.,3.06816841590428,9.57325067970064));
#30913=CARTESIAN_POINT('Ctrl Pts',(-8.,2.9146850890607,9.62594843092614));
#30914=CARTESIAN_POINT('Ctrl Pts',(-8.,2.75983355042631,9.67487206864313));
#30915=CARTESIAN_POINT('Ctrl Pts',(-8.,2.6037558201701,9.72001092048762));
#30916=CARTESIAN_POINT('Ctrl Pts',(0.711515937838069,-9.64233463315361,
5.55577575209881E-5));
#30917=CARTESIAN_POINT('Ctrl Pts',(0.710856866388953,-9.64235142088166,
0.053277087912501));
#30918=CARTESIAN_POINT('Ctrl Pts',(0.710197794939836,-9.64191990087921,
0.10649834290957));
#30919=CARTESIAN_POINT('Ctrl Pts',(0.70953872349072,-9.64103837930507,0.15971214088109));
#30920=CARTESIAN_POINT('Ctrl Pts',(0.689789202575776,-9.61462299021662,
1.75429952197757));
#30921=CARTESIAN_POINT('Ctrl Pts',(0.670039681660832,-9.18413243182588,
3.34219092899087));
#30922=CARTESIAN_POINT('Ctrl Pts',(0.650290160745888,-8.40151830542192,
4.73176597520196));
#30923=CARTESIAN_POINT('Ctrl Pts',(0.630540639830942,-7.61890417901792,
6.12134102141313));
#30924=CARTESIAN_POINT('Ctrl Pts',(0.610791118915997,-6.48416648460066,
7.31259970682207));
#30925=CARTESIAN_POINT('Ctrl Pts',(0.591041598001052,-5.13424259119184,
8.16178176230046));
#30926=CARTESIAN_POINT('Ctrl Pts',(0.571292077086108,-3.78431869778303,
9.01096381777884));
#30927=CARTESIAN_POINT('Ctrl Pts',(0.551542556171163,-2.21920860538266,
9.51806924332668));
#30928=CARTESIAN_POINT('Ctrl Pts',(0.531793035256218,-0.627786836456111,
9.62190242474063));
#30929=CARTESIAN_POINT('Ctrl Pts',(0.512043514341272,0.963634932470433,
9.72573560615459));
#30930=CARTESIAN_POINT('Ctrl Pts',(0.492293993426328,2.58136837792315,9.42629654343467));
#30931=CARTESIAN_POINT('Ctrl Pts',(0.472544472511382,4.03018885727291,8.75972049974441));
#30932=CARTESIAN_POINT('Ctrl Pts',(0.452794951596437,5.47900933662266,8.09314445605415));
#30933=CARTESIAN_POINT('Ctrl Pts',(0.433045430681492,6.75891684986946,7.05943143139355));
#30934=CARTESIAN_POINT('Ctrl Pts',(0.413295909766547,7.71545471159267,5.78332802334296));
#30935=CARTESIAN_POINT('Ctrl Pts',(0.393546388851601,8.67199257331588,4.50722461529236));
#30936=CARTESIAN_POINT('Ctrl Pts',(0.373796867936656,9.30516078351549,2.98873082385177));
#30937=CARTESIAN_POINT('Ctrl Pts',(0.354047347021711,9.53854992981817,1.41109525988503));
#30938=CARTESIAN_POINT('Ctrl Pts',(0.334297826106766,9.77193907612084,-0.166540304081665));
#30939=CARTESIAN_POINT('Ctrl Pts',(0.314548305191821,9.60554915852659,-1.8033176405745));
#30940=CARTESIAN_POINT('Ctrl Pts',(0.294798784276877,9.05945975514247,-3.3017137470004));
#30941=CARTESIAN_POINT('Ctrl Pts',(0.275049263361932,8.51337035175834,-4.80010985342633));
#30942=CARTESIAN_POINT('Ctrl Pts',(0.255299742446987,7.58758146258432,-6.16012472978531));
#30943=CARTESIAN_POINT('Ctrl Pts',(0.235550221532042,6.39381540689866,-7.2176345921584));
#30944=CARTESIAN_POINT('Ctrl Pts',(0.215800700617097,5.200049351213,-8.27514445453149));
#30945=CARTESIAN_POINT('Ctrl Pts',(0.196051179702152,3.7383061290157,-9.03014930291869));
#30946=CARTESIAN_POINT('Ctrl Pts',(0.176301658787207,2.18498591945131,-9.39153667969154));
#30947=CARTESIAN_POINT('Ctrl Pts',(0.156552137872262,0.631665709886971,
-9.75292405646439));
#30948=CARTESIAN_POINT('Ctrl Pts',(0.136802616957318,-1.01323148704445,
-9.7206939616229));
#30949=CARTESIAN_POINT('Ctrl Pts',(0.117053096042373,-2.55120283805044,
-9.29873586542844));
#30950=CARTESIAN_POINT('Ctrl Pts',(0.0973035751274285,-4.08917418905644,
-8.87677776923399));
#30951=CARTESIAN_POINT('Ctrl Pts',(0.0775540542124838,-5.52021969413699,
-8.06509167168657));
#30952=CARTESIAN_POINT('Ctrl Pts',(0.0578045332975393,-6.67164370855832,
-6.96163018734359));
#30953=CARTESIAN_POINT('Ctrl Pts',(0.0380550123825936,-7.8230677229797,
-5.85816870300055));
#30954=CARTESIAN_POINT('Ctrl Pts',(0.0183054914676481,-8.69487024674182,
-4.46293183186192));
#30955=CARTESIAN_POINT('Ctrl Pts',(-0.00144402944729742,-9.1818439329385,
-2.94429390937257));
#30956=CARTESIAN_POINT('Ctrl Pts',(-0.013790707018842,-9.48628205653607,
-1.99489706791769));
#30957=CARTESIAN_POINT('Ctrl Pts',(-0.0261373845903865,-9.6403178056493,
-0.997271483382048));
#30958=CARTESIAN_POINT('Ctrl Pts',(-0.0384840621619312,-9.6409393879154,
0.000166496178767295));
#30959=CARTESIAN_POINT('Ctrl Pts',(-8.,-2.60344811511687,9.71940883564398));
#30960=CARTESIAN_POINT('Ctrl Pts',(-7.98025047908506,-4.2115554043733,9.28866001522532));
#30961=CARTESIAN_POINT('Ctrl Pts',(-7.94075143725516,-7.20829614504029,
7.61418486945486));
#30962=CARTESIAN_POINT('Ctrl Pts',(-7.88150287451034,-9.96442823502186,
3.26156338357991));
#30963=CARTESIAN_POINT('Ctrl Pts',(-7.82225431176549,-10.3152149209058,
-1.87689719875276));
#30964=CARTESIAN_POINT('Ctrl Pts',(-7.76300574902067,-8.17655263057037,
-6.56303005806257));
#30965=CARTESIAN_POINT('Ctrl Pts',(-7.70375718627582,-4.06433342707358,
-9.66479172255802));
#30966=CARTESIAN_POINT('Ctrl Pts',(-7.644508623531,1.02878615653537,-10.4340771844272));
#30967=CARTESIAN_POINT('Ctrl Pts',(-7.58526006078616,5.87362828262073,-8.68494406353048));
#30968=CARTESIAN_POINT('Ctrl Pts',(-7.52601149804132,9.30082195115954,-4.83969619824767));
#30969=CARTESIAN_POINT('Ctrl Pts',(-7.46676293529649,10.483214281353,0.173665734501785));
#30970=CARTESIAN_POINT('Ctrl Pts',(-7.40751437255165,9.13541724029078,5.1450995797055));
#30971=CARTESIAN_POINT('Ctrl Pts',(-7.34826580980682,5.58273512973762,8.87473987601911));
#30972=CARTESIAN_POINT('Ctrl Pts',(-7.28901724706198,0.682625919309218,
10.4624057987323));
#30973=CARTESIAN_POINT('Ctrl Pts',(-7.22976868431715,-4.38223858668436,
9.52491001985317));
#30974=CARTESIAN_POINT('Ctrl Pts',(-7.17052012157231,-8.38942416699272,
6.28851997968158));
#30975=CARTESIAN_POINT('Ctrl Pts',(-7.11127155882747,-10.371772497116,1.53435894800687));
#30976=CARTESIAN_POINT('Ctrl Pts',(-7.05202299608265,-9.85083229519261,
-3.59012893362295));
#30977=CARTESIAN_POINT('Ctrl Pts',(-6.9927744333378,-6.95233545178506,-7.84811784659899));
#30978=CARTESIAN_POINT('Ctrl Pts',(-6.93352587059297,-2.37585136897494,
-10.2119171916642));
#30979=CARTESIAN_POINT('Ctrl Pts',(-6.87427730784814,2.77405849573116,-10.1110099229398));
#30980=CARTESIAN_POINT('Ctrl Pts',(-6.8150287451033,7.25443293930229,-7.56975065851036));
#30981=CARTESIAN_POINT('Ctrl Pts',(-6.75578018235847,9.98390711286757,-3.20148731676458));
#30982=CARTESIAN_POINT('Ctrl Pts',(-6.69653161961363,10.3037062860758,1.93947390886785));
#30983=CARTESIAN_POINT('Ctrl Pts',(-6.63728305686881,8.13664504012033,6.61233164437115));
#30984=CARTESIAN_POINT('Ctrl Pts',(-6.57803449412396,4.00575641567419,9.68926404911563));
#30985=CARTESIAN_POINT('Ctrl Pts',(-6.51878593137913,-1.09194519850991,
10.4276353006677));
#30986=CARTESIAN_POINT('Ctrl Pts',(-6.45953736863429,-5.92609938437677,
8.64923513176283));
#30987=CARTESIAN_POINT('Ctrl Pts',(-6.40028880588946,-9.32995445315455,
4.78329093624652));
#30988=CARTESIAN_POINT('Ctrl Pts',(-6.34104024314462,-10.4819698630527,
-0.237128802024965));
#30989=CARTESIAN_POINT('Ctrl Pts',(-6.28179168039979,-9.10409988500852,
-5.20031610215367));
#30990=CARTESIAN_POINT('Ctrl Pts',(-6.22254311765495,-5.52890158316907,
-8.90837637071521));
#30991=CARTESIAN_POINT('Ctrl Pts',(-6.16329455491012,-0.61927020154201,
-10.4663473426058));
#30992=CARTESIAN_POINT('Ctrl Pts',(-6.10404599216529,4.43982570388255,-9.49820351423256));
#30993=CARTESIAN_POINT('Ctrl Pts',(-6.04479742942044,8.42734343078316,-6.23761212149772));
#30994=CARTESIAN_POINT('Ctrl Pts',(-5.98554886667563,10.3808720045808,-1.47153617119417));
#30995=CARTESIAN_POINT('Ctrl Pts',(-5.92630030393077,9.82891575620613,3.64970373263731));
#30996=CARTESIAN_POINT('Ctrl Pts',(-5.86705174118595,6.90469258895211,7.89006606630713));
#30997=CARTESIAN_POINT('Ctrl Pts',(-5.80780317844112,2.31398105003217,10.2261143147686));
#30998=CARTESIAN_POINT('Ctrl Pts',(-5.74855461569627,-2.83522349381956,
10.094029424304));
#30999=CARTESIAN_POINT('Ctrl Pts',(-5.68930605295145,-7.3001300877402,7.5256908640133));
#31000=CARTESIAN_POINT('Ctrl Pts',(-5.63005749020659,-10.0031071321348,
3.14098232749819));
#31001=CARTESIAN_POINT('Ctrl Pts',(-5.57080892746178,-10.2917751393821,
-2.00182086087136));
#31002=CARTESIAN_POINT('Ctrl Pts',(-5.51156036471693,-8.09646237954581,
-6.66147275121817));
#31003=CARTESIAN_POINT('Ctrl Pts',(-5.4523118019721,-3.94702056424182,-9.71333881546786));
#31004=CARTESIAN_POINT('Ctrl Pts',(-5.39306323922727,1.15505799604341,-10.420833138689));
#31005=CARTESIAN_POINT('Ctrl Pts',(-5.33381467648243,5.97835648115395,-8.61319778380056));
#31006=CARTESIAN_POINT('Ctrl Pts',(-5.27456611373759,9.35874329001436,-4.72671622907851));
#31007=CARTESIAN_POINT('Ctrl Pts',(-5.21531755099276,10.480342084015,0.300586228304444));
#31008=CARTESIAN_POINT('Ctrl Pts',(-5.15606898824793,9.07244836417983,5.25534042264758));
#31009=CARTESIAN_POINT('Ctrl Pts',(-5.09682042550309,5.47486560219418,8.9416871403854));
#31010=CARTESIAN_POINT('Ctrl Pts',(-5.03757186275826,0.555891663852748,
10.4699048102971));
#31011=CARTESIAN_POINT('Ctrl Pts',(-4.97832330001342,-4.49725001357077,
9.47114906408194));
#31012=CARTESIAN_POINT('Ctrl Pts',(-4.91907473726859,-8.464953815877,6.18647550497794));
#31013=CARTESIAN_POINT('Ctrl Pts',(-4.85982617452375,-10.3895909763142,
1.40865951298154));
#31014=CARTESIAN_POINT('Ctrl Pts',(-4.80057761177892,-9.80663893921103,
-3.70914477940301));
#31015=CARTESIAN_POINT('Ctrl Pts',(-4.74132904903408,-6.85679662469408,
-7.93172505361893));
#31016=CARTESIAN_POINT('Ctrl Pts',(-4.68208048628925,-2.25202591260958,
-10.2399365997821));
#31017=CARTESIAN_POINT('Ctrl Pts',(-4.62283192354441,2.89628456575783,-10.0766789168245));
#31018=CARTESIAN_POINT('Ctrl Pts',(-4.56358336079958,7.34555964353492,-7.48135521158391));
#31019=CARTESIAN_POINT('Ctrl Pts',(-4.50433479805474,10.0219404799498,-3.08036220191168));
#31020=CARTESIAN_POINT('Ctrl Pts',(-4.44508623530991,10.2794667393936,2.0640944339644));
#31021=CARTESIAN_POINT('Ctrl Pts',(-4.38583767256508,8.0559829368491,6.71036967683738));
#31022=CARTESIAN_POINT('Ctrl Pts',(-4.32658910982024,3.88814003161556,9.73705753157345));
#31023=CARTESIAN_POINT('Ctrl Pts',(-4.2673405470754,-1.21812845399267,10.4136489929417));
#31024=CARTESIAN_POINT('Ctrl Pts',(-4.20809198433057,-6.03039443657531,
8.57684471224378));
#31025=CARTESIAN_POINT('Ctrl Pts',(-4.14884342158573,-9.3871890747578,4.66996826042431));
#31026=CARTESIAN_POINT('Ctrl Pts',(-4.08959485884091,-10.4783301397828,
-0.364032636370266));
#31027=CARTESIAN_POINT('Ctrl Pts',(-4.03034629609606,-9.04046428560539,
-5.31017210449113));
#31028=CARTESIAN_POINT('Ctrl Pts',(-3.97109773335123,-5.42062893570726,
-8.9746701454703));
#31029=CARTESIAN_POINT('Ctrl Pts',(-3.9118491706064,-0.492492749516077,
-10.4730784953755));
#31030=CARTESIAN_POINT('Ctrl Pts',(-3.85260060786156,4.5545094730156,-9.4437474414998));
#31031=CARTESIAN_POINT('Ctrl Pts',(-3.79335204511673,8.50225391141831,-6.13511211832306));
#31032=CARTESIAN_POINT('Ctrl Pts',(-3.73410348237189,10.3979291094031,-1.34573121924465));
#31033=CARTESIAN_POINT('Ctrl Pts',(-3.67485491962706,9.78400265213786,3.76844986454401));
#31034=CARTESIAN_POINT('Ctrl Pts',(-3.61560635688222,6.80864931915254,7.97309329729851));
#31035=CARTESIAN_POINT('Ctrl Pts',(-3.55635779413739,2.18998822540255,10.2533835318504));
#31036=CARTESIAN_POINT('Ctrl Pts',(-3.49710923139255,-2.95723947210302,
10.0589590407387));
#31037=CARTESIAN_POINT('Ctrl Pts',(-3.43786066864772,-7.39071994205252,
7.43674532418379));
#31038=CARTESIAN_POINT('Ctrl Pts',(-3.37861210590288,-10.040406465639,3.01962916322129));
#31039=CARTESIAN_POINT('Ctrl Pts',(-3.31936354315805,-10.2667815374515,
-2.1262923460494));
#31040=CARTESIAN_POINT('Ctrl Pts',(-3.26011498041321,-8.01520819574961,
-6.75902062856823));
#31041=CARTESIAN_POINT('Ctrl Pts',(-3.20086641766838,-3.82911697615253,
-9.76041932816225));
#31042=CARTESIAN_POINT('Ctrl Pts',(-3.14161785492354,1.28115426048353,-10.4060831266845));
#31043=CARTESIAN_POINT('Ctrl Pts',(-3.08236929217871,6.08221134313651,-8.54017724968541));
#31044=CARTESIAN_POINT('Ctrl Pts',(-3.02312072943387,9.41529076468844,-4.61304911040355));
#31045=CARTESIAN_POINT('Ctrl Pts',(-2.96387216668904,10.4759341041022,0.427465700532903));
#31046=CARTESIAN_POINT('Ctrl Pts',(-2.9046236039442,9.00814882168857,5.36480913779172));
#31047=CARTESIAN_POINT('Ctrl Pts',(-2.84537504119937,5.36619357179512,9.00732417694884));
#31048=CARTESIAN_POINT('Ctrl Pts',(-2.78612647845453,0.429075782469587,
10.4758682815087));
#31049=CARTESIAN_POINT('Ctrl Pts',(-2.7268779157097,-4.61160198332664,9.41599965091337));
#31050=CARTESIAN_POINT('Ctrl Pts',(-2.66762935296486,-8.5392423501426,6.08352384429894));
#31051=CARTESIAN_POINT('Ctrl Pts',(-2.60838079022003,-10.4058860982068,
1.28275359666941));
#31052=CARTESIAN_POINT('Ctrl Pts',(-2.54913222747519,-9.7610077247375,-3.82761681418572));
#31053=CARTESIAN_POINT('Ctrl Pts',(-2.48988366473036,-6.76025243720484,
-8.01416928096036));
#31054=CARTESIAN_POINT('Ctrl Pts',(-2.43063510198552,-2.12787026245138,
-10.2664546180655));
#31055=CARTESIAN_POINT('Ctrl Pts',(-2.37138653924069,3.01808597850499,-10.0408704455826));
#31056=CARTESIAN_POINT('Ctrl Pts',(-2.31213797649586,7.43560932790665,-7.39186283702356));
#31057=CARTESIAN_POINT('Ctrl Pts',(-2.25288941375102,10.0585044123173,-2.95878543764436));
#31058=CARTESIAN_POINT('Ctrl Pts',(-2.19364085100618,10.2537199985417,2.18841231721289));
#31059=CARTESIAN_POINT('Ctrl Pts',(-2.13439228826135,7.97413965087761,6.80742382307171));
#31060=CARTESIAN_POINT('Ctrl Pts',(-2.07514372551652,3.76995356138932,9.78342334888923));
#31061=CARTESIAN_POINT('Ctrl Pts',(-2.01589516277168,-1.34413310525547,
10.3981358172501));
#31062=CARTESIAN_POINT('Ctrl Pts',(-1.95664660002685,-6.1338053014481,8.50319674020009));
#31063=CARTESIAN_POINT('Ctrl Pts',(-1.89739803728201,-9.44304732971672,
4.5559608654325));
#31064=CARTESIAN_POINT('Ctrl Pts',(-1.83814947453718,-10.4731540648018,
-0.490883095603427));
#31065=CARTESIAN_POINT('Ctrl Pts',(-1.77890091179234,-8.97550315697813,
-5.41924951978578));
#31066=CARTESIAN_POINT('Ctrl Pts',(-1.71965234904751,-5.31156150582896,
-9.03964803786181));
#31067=CARTESIAN_POINT('Ctrl Pts',(-1.66040378630267,-0.365643087312114,
-10.4782740664349));
#31068=CARTESIAN_POINT('Ctrl Pts',(-1.60115522355784,4.66852545173299,-9.38790670943975));
#31069=CARTESIAN_POINT('Ctrl Pts',(-1.541906660813,8.57591777620947,-6.03171257391441));
#31070=CARTESIAN_POINT('Ctrl Pts',(-1.48265809806816,10.4134616510556,-1.2197289537503));
#31071=CARTESIAN_POINT('Ctrl Pts',(-1.42340953532333,9.73765499990719,3.88664345951686));
#31072=CARTESIAN_POINT('Ctrl Pts',(-1.3641609725785,6.71160775287686,8.05495149893194));
#31073=CARTESIAN_POINT('Ctrl Pts',(-1.30491240983366,2.06567430073889,10.2791493792964));
#31074=CARTESIAN_POINT('Ctrl Pts',(-1.24566384708883,-3.07882185458713,
10.022413794408));
#31075=CARTESIAN_POINT('Ctrl Pts',(-1.18641528434399,-7.48022615564147,
7.34670939530617));
#31076=CARTESIAN_POINT('Ctrl Pts',(-1.12716672159916,-10.07623365659,2.89783325545567));
#31077=CARTESIAN_POINT('Ctrl Pts',(-1.06791815885432,-10.2402826014452,
-2.25045207039839));
#31078=CARTESIAN_POINT('Ctrl Pts',(-1.00866959610949,-7.93277880763296,
-6.85557748609057));
#31079=CARTESIAN_POINT('Ctrl Pts',(-0.949421033364655,-3.7106519560076,
-9.80606875052385));
#31080=CARTESIAN_POINT('Ctrl Pts',(-0.890172470619817,1.40706267976922,
-10.3898073559533));
#31081=CARTESIAN_POINT('Ctrl Pts',(-0.830923907874984,6.18517442029282,
-8.46590453933774));
#31082=CARTESIAN_POINT('Ctrl Pts',(-0.771675345130147,9.47045775240396,
-4.49870561812545));
#31083=CARTESIAN_POINT('Ctrl Pts',(-0.712426782385315,10.4699901237859,
0.554282496966878));
#31084=CARTESIAN_POINT('Ctrl Pts',(-0.65317821964048,8.94252848812691,5.47349125491902));
#31085=CARTESIAN_POINT('Ctrl Pts',(-0.593929656895644,5.25673474038977,
9.07164054335094));
#31086=CARTESIAN_POINT('Ctrl Pts',(-0.53468109415081,0.302196989220137,
10.4802957619713));
#31087=CARTESIAN_POINT('Ctrl Pts',(-0.475432531405974,-4.72527779166189,
9.35946964684205));
#31088=CARTESIAN_POINT('Ctrl Pts',(-0.41618396866114,-8.61227884524871,
5.97968020636365));
#31089=CARTESIAN_POINT('Ctrl Pts',(-0.356935405916305,-10.4206554902685,
1.15665960068344));
#31090=CARTESIAN_POINT('Ctrl Pts',(-0.29768684317147,-9.71394533364604,
-3.94552763682723));
#31091=CARTESIAN_POINT('Ctrl Pts',(-0.238438280426636,-6.66271704930368,
-8.09543845639));
#31092=CARTESIAN_POINT('Ctrl Pts',(-0.1791897176818,-2.00340262005729,-10.2914673500501));
#31093=CARTESIAN_POINT('Ctrl Pts',(-0.119941154936964,3.13944487393184,
-10.0035897640602));
#31094=CARTESIAN_POINT('Ctrl Pts',(-0.0606925921921299,7.52456878997794,
-7.3012866535828));
#31095=CARTESIAN_POINT('Ctrl Pts',(-0.00144402944729414,10.0935935482191,
-2.83677485203218));
#31096=CARTESIAN_POINT('Ctrl Pts',(0.0578045332975393,10.2264698394132,
2.3124093336654));
#31097=CARTESIAN_POINT('Ctrl Pts',(0.117053096042374,7.89112718079254,6.90347984831441));
#31098=CARTESIAN_POINT('Ctrl Pts',(0.176301658787208,3.65121433633638,9.82835471108965));
#31099=CARTESIAN_POINT('Ctrl Pts',(0.235550221532044,-1.46994068227644,
10.3810980324261));
#31100=CARTESIAN_POINT('Ctrl Pts',(0.294798784276879,-6.23631680707128,
8.42830204429616));
#31101=CARTESIAN_POINT('Ctrl Pts',(0.354047347021714,-9.4975210465794,4.44128540887));
#31102=CARTESIAN_POINT('Ctrl Pts',(0.413295909766549,-10.4664423611608,
-0.617661468019164));
#31103=CARTESIAN_POINT('Ctrl Pts',(0.472544472511383,-8.90922609310004,
-5.52753257240065));
#31104=CARTESIAN_POINT('Ctrl Pts',(0.531793035256219,-5.20171515149495,
-9.10330010082978));
#31105=CARTESIAN_POINT('Ctrl Pts',(0.591041598001052,-0.23874007198555,
-10.4819341046316));
#31106=CARTESIAN_POINT('Ctrl Pts',(0.650290160745889,4.78185742115312,-9.33068794050316));
#31107=CARTESIAN_POINT('Ctrl Pts',(0.709538723490722,8.64832326230869,-5.92743167035388));
#31108=CARTESIAN_POINT('Ctrl Pts',(0.768787286235557,10.4274692096169,-1.09354201610874));
#31109=CARTESIAN_POINT('Ctrl Pts',(0.828035848980392,9.68987600895932,4.00425592589309));
#31110=CARTESIAN_POINT('Ctrl Pts',(0.887284411725228,6.61358904227201,8.1356504120078));
#31111=CARTESIAN_POINT('Ctrl Pts',(0.946532974470063,1.9410441333556,10.3033660965346));
#31112=CARTESIAN_POINT('Ctrl Pts',(1.0057815372149,-3.19992697648555,9.98448014714238));
#31113=CARTESIAN_POINT('Ctrl Pts',(1.06503009995973,-7.56868573973501,7.25543921015781));
#31114=CARTESIAN_POINT('Ctrl Pts',(1.12427866270457,-10.1104842470233,2.77592039631992));
#31115=CARTESIAN_POINT('Ctrl Pts',(1.1835272254494,-10.2124968952733,-2.37492141025147));
#31116=CARTESIAN_POINT('Ctrl Pts',(1.22302626727929,-8.63654184006421,-5.42462430472119));
#31117=CARTESIAN_POINT('Ctrl Pts',(1.24277578819424,-7.53281147710298,-6.67095206495486));
#31118=CARTESIAN_POINT('Ctrl Pts',(-8.08092526273141,-2.56718148514231,
9.58401523906448));
#31119=CARTESIAN_POINT('Ctrl Pts',(-8.06117574181647,-4.15288747065075,
9.15926684861076));
#31120=CARTESIAN_POINT('Ctrl Pts',(-8.02167669998656,-7.10788292477239,
7.50811752606706));
#31121=CARTESIAN_POINT('Ctrl Pts',(-7.96242813724176,-9.82562146195453,
3.21612905681762));
#31122=CARTESIAN_POINT('Ctrl Pts',(-7.9031795744969,-10.1715216087662,-1.85075158985345));
#31123=CARTESIAN_POINT('Ctrl Pts',(-7.84393101175209,-8.06265137515507,
-6.47160554253427));
#31124=CARTESIAN_POINT('Ctrl Pts',(-7.78468244900723,-4.0077163292958,-9.53015895490345));
#31125=CARTESIAN_POINT('Ctrl Pts',(-7.72543388626241,1.01445492917372,-10.288728093667));
#31126=CARTESIAN_POINT('Ctrl Pts',(-7.66618532351757,5.79180729210547,-8.56396079873138));
#31127=CARTESIAN_POINT('Ctrl Pts',(-7.60693676077273,9.17125936598514,-4.77227811905034));
#31128=CARTESIAN_POINT('Ctrl Pts',(-7.54768819802789,10.3371806995511,0.171246530947913));
#31129=CARTESIAN_POINT('Ctrl Pts',(-7.48843963528308,9.00815878071438,5.07342716128625));
#31130=CARTESIAN_POINT('Ctrl Pts',(-7.42919107253822,5.50496634762878,8.75111271197646));
#31131=CARTESIAN_POINT('Ctrl Pts',(-7.3699425097934,0.673116783527759,10.3166620838708));
#31132=CARTESIAN_POINT('Ctrl Pts',(-7.31069394704856,-4.32119299704472,
9.39222583643303));
#31133=CARTESIAN_POINT('Ctrl Pts',(-7.25144538430372,-8.27255756220144,
6.20091945257043));
#31134=CARTESIAN_POINT('Ctrl Pts',(-7.19219682155889,-10.2272913249547,
1.51298497558452));
#31135=CARTESIAN_POINT('Ctrl Pts',(-7.13294825881406,-9.71360793964782,
-3.54011761331254));
#31136=CARTESIAN_POINT('Ctrl Pts',(-7.07369969606921,-6.85548782274077,
-7.73879176313041));
#31137=CARTESIAN_POINT('Ctrl Pts',(-7.0144511333244,-2.34275521392854,-10.0696628406093));
#31138=CARTESIAN_POINT('Ctrl Pts',(-6.95520257057954,2.73541522398385,-9.9701612333058));
#31139=CARTESIAN_POINT('Ctrl Pts',(-6.89595400783472,7.15337702289769,-7.46430229388277));
#31140=CARTESIAN_POINT('Ctrl Pts',(-6.83670544508987,9.84482899455965,-3.15688986340601));
#31141=CARTESIAN_POINT('Ctrl Pts',(-6.77745688234505,10.1601732918617,1.91245659202953));
#31142=CARTESIAN_POINT('Ctrl Pts',(-6.71820831960021,8.02329970660245,6.5202203464263));
#31143=CARTESIAN_POINT('Ctrl Pts',(-6.65895975685538,3.94995530911404,9.55429037633348));
#31144=CARTESIAN_POINT('Ctrl Pts',(-6.59971119411054,-1.07673415119273,
10.2823759468273));
#31145=CARTESIAN_POINT('Ctrl Pts',(-6.54046263136571,-5.84354745936712,
8.52874930058177));
#31146=CARTESIAN_POINT('Ctrl Pts',(-6.48121406862087,-9.19998604553876,
4.71665859529904));
#31147=CARTESIAN_POINT('Ctrl Pts',(-6.42196550587603,-10.3359536162835,
-0.233825543369873));
#31148=CARTESIAN_POINT('Ctrl Pts',(-6.36271694313121,-8.97727768338141,
-5.12787450489945));
#31149=CARTESIAN_POINT('Ctrl Pts',(-6.30346838038635,-5.45188271472368,
-8.78428064257877));
#31150=CARTESIAN_POINT('Ctrl Pts',(-6.24421981764154,-0.610643625455016,
-10.3205487211332));
#31151=CARTESIAN_POINT('Ctrl Pts',(-6.18497125489669,4.37797791247879,-9.3658913585673));
#31152=CARTESIAN_POINT('Ctrl Pts',(-6.12572269215187,8.30994860194132,-6.15072075253911));
#31153=CARTESIAN_POINT('Ctrl Pts',(-6.06647412940703,10.2362640741913,-1.45103733447644));
#31154=CARTESIAN_POINT('Ctrl Pts',(-6.00722556666219,9.69199670308129,3.59886252169872));
#31155=CARTESIAN_POINT('Ctrl Pts',(-5.94797700391735,6.80850863592549,7.78015563450705));
#31156=CARTESIAN_POINT('Ctrl Pts',(-5.88872844117253,2.28174676273358,10.0836621945293));
#31157=CARTESIAN_POINT('Ctrl Pts',(-5.82947987842768,-2.79572817960588,
9.9534172769146));
#31158=CARTESIAN_POINT('Ctrl Pts',(-5.77023131568286,-7.19843759956617,
7.42085626243881));
#31159=CARTESIAN_POINT('Ctrl Pts',(-5.71098275293802,-9.86376155315033,
3.09722772253158));
#31160=CARTESIAN_POINT('Ctrl Pts',(-5.65173419019319,-10.1484083487808,
-1.97393503667728));
#31161=CARTESIAN_POINT('Ctrl Pts',(-5.59248562744834,-7.98367679971535,
-6.56867690637251));
#31162=CARTESIAN_POINT('Ctrl Pts',(-5.53323706470353,-3.8920376615774,-9.57802977566305));
#31163=CARTESIAN_POINT('Ctrl Pts',(-5.47398850195867,1.1389677729664,-10.2756685405266));
#31164=CARTESIAN_POINT('Ctrl Pts',(-5.41473993921385,5.89507660278836,-8.49321396115051));
#31165=CARTESIAN_POINT('Ctrl Pts',(-5.35549137646901,9.22837384729142,-4.66087198679098));
#31166=CARTESIAN_POINT('Ctrl Pts',(-5.29624281372418,10.3343485125815,0.29639899313195));
#31167=CARTESIAN_POINT('Ctrl Pts',(-5.23699425097934,8.9460670755048,5.18213232397573));
#31168=CARTESIAN_POINT('Ctrl Pts',(-5.1777456882345,5.39859946737001,8.81712738557956));
#31169=CARTESIAN_POINT('Ctrl Pts',(-5.11849712548967,0.548147965346974,
10.3240566324828));
#31170=CARTESIAN_POINT('Ctrl Pts',(-5.05924856274483,-4.43460228834889,
9.33921378311876));
#31171=CARTESIAN_POINT('Ctrl Pts',(-5.,-8.34703506573574,6.10029648082801));
#31172=CARTESIAN_POINT('Ctrl Pts',(-4.94075143725517,-10.2448615886467,
1.38903656254868));
#31173=CARTESIAN_POINT('Ctrl Pts',(-4.88150287451033,-9.67003020726149,
-3.65747554103578));
#31174=CARTESIAN_POINT('Ctrl Pts',(-4.8222543117655,-6.76127987344612,-7.82123430256102));
#31175=CARTESIAN_POINT('Ctrl Pts',(-4.76300574902066,-2.22065467459968,
-10.0972919319392));
#31176=CARTESIAN_POINT('Ctrl Pts',(-4.70375718627583,2.85593865679291,-9.93630846598779));
#31177=CARTESIAN_POINT('Ctrl Pts',(-4.64450862353099,7.24323431121841,-7.37713821582688));
#31178=CARTESIAN_POINT('Ctrl Pts',(-4.58526006078616,9.88233254810626,-3.03745204921238));
#31179=CARTESIAN_POINT('Ctrl Pts',(-4.52601149804132,10.1362714076301,2.03534112459961));
#31180=CARTESIAN_POINT('Ctrl Pts',(-4.46676293529649,7.94376124494917,6.61689268659152));
#31181=CARTESIAN_POINT('Ctrl Pts',(-4.40751437255165,3.83397734828913,9.60141808460764));
#31182=CARTESIAN_POINT('Ctrl Pts',(-4.34826580980682,-1.20115964495595,
10.268584471579));
#31183=CARTESIAN_POINT('Ctrl Pts',(-4.28901724706198,-5.94638965754321,
8.45736729622688));
#31184=CARTESIAN_POINT('Ctrl Pts',(-4.22976868431715,-9.25642337572245,
4.60491453036902));
#31185=CARTESIAN_POINT('Ctrl Pts',(-4.17052012157231,-10.3323645951943,
-0.358961578166624));
#31186=CARTESIAN_POINT('Ctrl Pts',(-4.11127155882748,-8.91452854248819,
-5.23620018790229));
#31187=CARTESIAN_POINT('Ctrl Pts',(-4.05202299608264,-5.34511833009956,
-8.849650929831));
#31188=CARTESIAN_POINT('Ctrl Pts',(-3.99277443333781,-0.485632212442896,
-10.3271861073994));
#31189=CARTESIAN_POINT('Ctrl Pts',(-3.93352587059297,4.49106411037733,-9.31219387143038));
#31190=CARTESIAN_POINT('Ctrl Pts',(-3.87427730784814,8.38381556238237,-6.04964859794188));
#31191=CARTESIAN_POINT('Ctrl Pts',(-3.8150287451033,10.2530835696273,-1.32698487439137));
#31192=CARTESIAN_POINT('Ctrl Pts',(-3.75578018235847,9.64770924886438,3.71595449272479));
#31193=CARTESIAN_POINT('Ctrl Pts',(-3.69653161961364,6.713803270925,7.86202627710832));
#31194=CARTESIAN_POINT('Ctrl Pts',(-3.6372830568688,2.15948118661882,10.1105515451564));
#31195=CARTESIAN_POINT('Ctrl Pts',(-3.57803449412396,-2.91604444729796,
9.91883543184418));
#31196=CARTESIAN_POINT('Ctrl Pts',(-3.51878593137913,-7.2877655164092,7.33314975440033));
#31197=CARTESIAN_POINT('Ctrl Pts',(-3.45953736863429,-9.90054129837521,
2.97756503569476));
#31198=CARTESIAN_POINT('Ctrl Pts',(-3.40028880588946,-10.1237629134634,
-2.09667260548911));
#31199=CARTESIAN_POINT('Ctrl Pts',(-3.34104024314462,-7.90355450535475,
-6.66486591939489));
#31200=CARTESIAN_POINT('Ctrl Pts',(-3.28179168039979,-3.77577649753992,
-9.62445444600628));
#31201=CARTESIAN_POINT('Ctrl Pts',(-3.22254311765495,1.26330748749216,-10.2611239995758));
#31202=CARTESIAN_POINT('Ctrl Pts',(-3.16329455491012,5.99748474269926,-8.42121061984051));
#31203=CARTESIAN_POINT('Ctrl Pts',(-3.10404599216528,9.28413360266045,-4.54878827717624));
#31204=CARTESIAN_POINT('Ctrl Pts',(-3.04479742942045,10.3300019368408,0.421511005181756));
#31205=CARTESIAN_POINT('Ctrl Pts',(-2.98554886667561,8.88266324040311,5.29007611478477));
#31206=CARTESIAN_POINT('Ctrl Pts',(-2.92630030393078,5.29144126330465,8.88185008315394));
#31207=CARTESIAN_POINT('Ctrl Pts',(-2.86705174118594,0.423098658307396,
10.3299370311713));
#31208=CARTESIAN_POINT('Ctrl Pts',(-2.80780317844112,-4.54736130891176,
9.28483261393749));
#31209=CARTESIAN_POINT('Ctrl Pts',(-2.74855461569627,-8.42028874366297,
5.99877896041916));
#31210=CARTESIAN_POINT('Ctrl Pts',(-2.68930605295144,-10.2609297157501,
1.26488454455777));
#31211=CARTESIAN_POINT('Ctrl Pts',(-2.63005749020661,-9.62503464608216,
-3.77429723317373));
#31212=CARTESIAN_POINT('Ctrl Pts',(-2.57080892746177,-6.66608056865438,
-7.90253006288704));
#31213=CARTESIAN_POINT('Ctrl Pts',(-2.51156036471693,-2.09822854115333,
-10.1234405481395));
#31214=CARTESIAN_POINT('Ctrl Pts',(-2.4523118019721,2.97604334789586,-9.90099881497165));
#31215=CARTESIAN_POINT('Ctrl Pts',(-2.39306323922727,7.33202958281215,-7.2888924905909));
#31216=CARTESIAN_POINT('Ctrl Pts',(-2.33381467648243,9.91838713650106,-2.91756887718436));
#31217=CARTESIAN_POINT('Ctrl Pts',(-2.2745661137376,10.1108833247894,2.15792723119204));
#31218=CARTESIAN_POINT('Ctrl Pts',(-2.21531755099276,7.86305805474182,6.71259484628595));
#31219=CARTESIAN_POINT('Ctrl Pts',(-2.15606898824793,3.71743724272782,9.64713801544299));
#31220=CARTESIAN_POINT('Ctrl Pts',(-2.09682042550309,-1.325409022497,10.2532873979865));
#31221=CARTESIAN_POINT('Ctrl Pts',(-2.03757186275826,-6.04835998532599,
8.38474525734275));
#31222=CARTESIAN_POINT('Ctrl Pts',(-1.97832330001343,-9.31150351236521,
4.49249528456464));
#31223=CARTESIAN_POINT('Ctrl Pts',(-1.91907473726858,-10.3272606241262,
-0.484044981378821));
#31224=CARTESIAN_POINT('Ctrl Pts',(-1.85982617452376,-8.85047233729729,
-5.34375812975856));
#31225=CARTESIAN_POINT('Ctrl Pts',(-1.80057761177891,-5.23757023456047,
-8.9137236652631));
#31226=CARTESIAN_POINT('Ctrl Pts',(-1.74132904903408,-0.360549595157115,
-10.3323093029611));
#31227=CARTESIAN_POINT('Ctrl Pts',(-1.68208048628925,4.60349182033403,-9.25713101358854));
#31228=CARTESIAN_POINT('Ctrl Pts',(-1.62283192354441,8.45645327262435,-5.94768943292654));
#31229=CARTESIAN_POINT('Ctrl Pts',(-1.56358336079958,10.2683997394084,-1.20273784938449));
#31230=CARTESIAN_POINT('Ctrl Pts',(-1.50433479805474,9.60200723007033,3.83250162378335));
#31231=CARTESIAN_POINT('Ctrl Pts',(-1.44508623530991,6.61811351594752,7.94274417519902));
#31232=CARTESIAN_POINT('Ctrl Pts',(-1.38583767256507,2.0368989834672,10.1359584684318));
#31233=CARTESIAN_POINT('Ctrl Pts',(-1.32658910982024,-3.03593315927972,
9.88279926918536));
#31234=CARTESIAN_POINT('Ctrl Pts',(-1.26734054707541,-7.37602488789294,
7.2443680466835));
#31235=CARTESIAN_POINT('Ctrl Pts',(-1.20809198433057,-9.93586940833061,
2.8574657728877));
#31236=CARTESIAN_POINT('Ctrl Pts',(-1.14884342158574,-10.0976331137197,
-2.21910275637184));
#31237=CARTESIAN_POINT('Ctrl Pts',(-1.0895948588409,-7.8222733775397,-6.76007771772325));
#31238=CARTESIAN_POINT('Ctrl Pts',(-1.03034629609607,-3.65896172232424,
-9.66946796143364));
#31239=CARTESIAN_POINT('Ctrl Pts',(-0.971097733351229,1.38746197358963,
-10.2450749540678));
#31240=CARTESIAN_POINT('Ctrl Pts',(-0.911849170606397,6.09901352055129,
-8.34797254540039));
#31241=CARTESIAN_POINT('Ctrl Pts',(-0.852600607861559,9.33853210157117,
-4.43603761599793));
#31242=CARTESIAN_POINT('Ctrl Pts',(-0.793352045116727,10.3241407575351,
0.546561214525285));
#31243=CARTESIAN_POINT('Ctrl Pts',(-0.734103482371892,8.81795701315387,
5.39724426506792));
#31244=CARTESIAN_POINT('Ctrl Pts',(-0.674854919627056,5.18350721855164,
8.94527050780554));
#31245=CARTESIAN_POINT('Ctrl Pts',(-0.615606356882222,0.297987315778273,
10.3343028358144));
#31246=CARTESIAN_POINT('Ctrl Pts',(-0.556357794137386,-4.65945358713783,
9.22909008580174));
#31247=CARTESIAN_POINT('Ctrl Pts',(-0.497109231392552,-8.49230782362366,
5.89638188820198));
#31248=CARTESIAN_POINT('Ctrl Pts',(-0.437860668647716,-10.2754933667894,
1.14054706688608));
#31249=CARTESIAN_POINT('Ctrl Pts',(-0.378612105902882,-9.57862784490375,
-3.89056553098446));
#31250=CARTESIAN_POINT('Ctrl Pts',(-0.319363543158048,-6.56990387110002,
-7.98266714004419));
#31251=CARTESIAN_POINT('Ctrl Pts',(-0.260114980413213,-1.97549476159458,
-10.1481048470248));
#31252=CARTESIAN_POINT('Ctrl Pts',(-0.200866417668376,3.09571168604639,
-9.86423746190218));
#31253=CARTESIAN_POINT('Ctrl Pts',(-0.141617854923542,7.4197498191524,-7.19957805418105));
#31254=CARTESIAN_POINT('Ctrl Pts',(-0.0823692921787063,9.95298747268358,
-2.79725792704241));
#31255=CARTESIAN_POINT('Ctrl Pts',(-0.0231207294338726,10.0840127666341,
2.28019694073663));
#31256=CARTESIAN_POINT('Ctrl Pts',(0.036127833310962,7.78120196742404,6.80731278904333));
#31257=CARTESIAN_POINT('Ctrl Pts',(0.0953763960557959,3.60035208234145,
9.69144347345206));
#31258=CARTESIAN_POINT('Ctrl Pts',(0.154624958800632,-1.44946407108565,
10.2364869534169));
#31259=CARTESIAN_POINT('Ctrl Pts',(0.213873521545467,-6.14944348214002,
8.31089386174798));
#31260=CARTESIAN_POINT('Ctrl Pts',(0.273122084290302,-9.36521839784525,
4.37941728344064));
#31261=CARTESIAN_POINT('Ctrl Pts',(0.332370647035137,-10.3206424160579,
-0.609057301959502));
#31262=CARTESIAN_POINT('Ctrl Pts',(0.391619209779971,-8.78511852813569,
-5.45053277458957));
#31263=CARTESIAN_POINT('Ctrl Pts',(0.450867772524806,-5.1292540651622,-8.97648904037991));
#31264=CARTESIAN_POINT('Ctrl Pts',(0.510116335269641,-0.235414367969966,
-10.3359183559853));
#31265=CARTESIAN_POINT('Ctrl Pts',(0.569364898014477,4.71524504940002,-9.20070931524018));
#31266=CARTESIAN_POINT('Ctrl Pts',(0.628613460759311,8.52785013367849,-5.84486118629469));
#31267=CARTESIAN_POINT('Ctrl Pts',(0.687862023504145,10.2822121694629,-1.07830872475579));
#31268=CARTESIAN_POINT('Ctrl Pts',(0.74711058624898,9.55489381143604,3.94847572150008));
#31269=CARTESIAN_POINT('Ctrl Pts',(0.806359148993816,6.52146022848571,8.02231893388788));
#31270=CARTESIAN_POINT('Ctrl Pts',(0.865607711738651,1.91400494292965,10.159837841239));
#31271=CARTESIAN_POINT('Ctrl Pts',(0.924856274483484,-3.15535125902531,
9.84539404633543));
#31272=CARTESIAN_POINT('Ctrl Pts',(0.98410483722832,-7.46325220967044,7.15436927616918));
#31273=CARTESIAN_POINT('Ctrl Pts',(1.04335339997316,-9.96964288017544,2.73725118786993));
#31274=CARTESIAN_POINT('Ctrl Pts',(1.10260196271799,-10.0702344688141,-2.34183820974359));
#31275=CARTESIAN_POINT('Ctrl Pts',(1.14210100454788,-8.51623282935078,-5.34905804270582));
#31276=CARTESIAN_POINT('Ctrl Pts',(1.16185052546282,-7.42787768375332,-6.5780241710925));
#31277=CARTESIAN_POINT('Ctrl Pts',(-8.16185052546282,-2.53091485516775,
9.44862164248498));
#31278=CARTESIAN_POINT('Ctrl Pts',(-8.14210100454788,-4.09421953692821,
9.02987368199619));
#31279=CARTESIAN_POINT('Ctrl Pts',(-8.10260196271799,-7.00746970450451,
7.40205018267925));
#31280=CARTESIAN_POINT('Ctrl Pts',(-8.04335339997316,-9.68681468888719,
3.17069473005534));
#31281=CARTESIAN_POINT('Ctrl Pts',(-7.98410483722832,-10.0278282966267,
-1.82460598095417));
#31282=CARTESIAN_POINT('Ctrl Pts',(-7.92485627448349,-7.94875011973976,
-6.38018102700592));
#31283=CARTESIAN_POINT('Ctrl Pts',(-7.86560771173864,-3.95109923151803,
-9.3955261872489));
#31284=CARTESIAN_POINT('Ctrl Pts',(-7.80635914899382,1.00012370181206,-10.1433790029068));
#31285=CARTESIAN_POINT('Ctrl Pts',(-7.74711058624898,5.70998630159022,-8.44297753393233));
#31286=CARTESIAN_POINT('Ctrl Pts',(-7.68786202350414,9.04169678081072,-4.70486003985297));
#31287=CARTESIAN_POINT('Ctrl Pts',(-7.62861346075931,10.1911471177493,0.168827327394019));
#31288=CARTESIAN_POINT('Ctrl Pts',(-7.56936489801448,8.88090032113799,5.00175474286701));
#31289=CARTESIAN_POINT('Ctrl Pts',(-7.51011633526964,5.42719756551993,8.6274855479338));
#31290=CARTESIAN_POINT('Ctrl Pts',(-7.45086777252481,0.663607647746304,
10.1709183690093));
#31291=CARTESIAN_POINT('Ctrl Pts',(-7.39161920977997,-4.26014740740508,
9.25954165301287));
#31292=CARTESIAN_POINT('Ctrl Pts',(-7.33237064703514,-8.15569095741015,
6.11331892545928));
#31293=CARTESIAN_POINT('Ctrl Pts',(-7.27312208429031,-10.0828101527934,
1.49161100316218));
#31294=CARTESIAN_POINT('Ctrl Pts',(-7.21387352154547,-9.57638358410301,
-3.49010629300211));
#31295=CARTESIAN_POINT('Ctrl Pts',(-7.15462495880062,-6.75864019369647,
-7.62946567966184));
#31296=CARTESIAN_POINT('Ctrl Pts',(-7.0953763960558,-2.30965905888213,-9.92740848955444));
#31297=CARTESIAN_POINT('Ctrl Pts',(-7.03612783331096,2.69677195223654,-9.82931254367178));
#31298=CARTESIAN_POINT('Ctrl Pts',(-6.97687927056613,7.0523211064931,-7.35885392925516));
#31299=CARTESIAN_POINT('Ctrl Pts',(-6.91763070782129,9.70575087625173,-3.11229241004746));
#31300=CARTESIAN_POINT('Ctrl Pts',(-6.85838214507646,10.0166402976476,1.88543927519122));
#31301=CARTESIAN_POINT('Ctrl Pts',(-6.79913358233163,7.90995437308458,6.42810904848144));
#31302=CARTESIAN_POINT('Ctrl Pts',(-6.73988501958678,3.89415420255387,9.41931670355132));
#31303=CARTESIAN_POINT('Ctrl Pts',(-6.68063645684196,-1.06152310387555,
10.1371165929868));
#31304=CARTESIAN_POINT('Ctrl Pts',(-6.62138789409712,-5.76099553435745,
8.4082634694007));
#31305=CARTESIAN_POINT('Ctrl Pts',(-6.56213933135228,-9.07001763792296,
4.65002625435157));
#31306=CARTESIAN_POINT('Ctrl Pts',(-6.50289076860745,-10.1899373695142,
-0.230522284714781));
#31307=CARTESIAN_POINT('Ctrl Pts',(-6.44364220586261,-8.85045548175431,
-5.05543290764522));
#31308=CARTESIAN_POINT('Ctrl Pts',(-6.38439364311778,-5.3748638462783,-8.66018491444234));
#31309=CARTESIAN_POINT('Ctrl Pts',(-6.32514508037295,-0.602017049368022,
-10.1747500996605));
#31310=CARTESIAN_POINT('Ctrl Pts',(-6.26589651762811,4.31613012107503,-9.23357920290205));
#31311=CARTESIAN_POINT('Ctrl Pts',(-6.20664795488327,8.19255377309947,-6.06382938358051));
#31312=CARTESIAN_POINT('Ctrl Pts',(-6.14739939213844,10.0916561438018,-1.4305384977587));
#31313=CARTESIAN_POINT('Ctrl Pts',(-6.0881508293936,9.55507764995644,3.54802131076013));
#31314=CARTESIAN_POINT('Ctrl Pts',(-6.02890226664877,6.71232468289887,7.67024520270696));
#31315=CARTESIAN_POINT('Ctrl Pts',(-5.96965370390394,2.24951247543498,9.9412100742901));
#31316=CARTESIAN_POINT('Ctrl Pts',(-5.91040514115909,-2.75623286539221,
9.81280512952515));
#31317=CARTESIAN_POINT('Ctrl Pts',(-5.85115657841427,-7.09674511139212,
7.31602166086433));
#31318=CARTESIAN_POINT('Ctrl Pts',(-5.79190801566943,-9.72441597416585,
3.05347311756495));
#31319=CARTESIAN_POINT('Ctrl Pts',(-5.7326594529246,-10.0050415581794,-1.94604921248318));
#31320=CARTESIAN_POINT('Ctrl Pts',(-5.67341089017976,-7.87089121988491,
-6.47588106152688));
#31321=CARTESIAN_POINT('Ctrl Pts',(-5.61416232743493,-3.83705475891298,
-9.44272073585823));
#31322=CARTESIAN_POINT('Ctrl Pts',(-5.55491376469009,1.12287754988938,-10.1305039423643));
#31323=CARTESIAN_POINT('Ctrl Pts',(-5.49566520194526,5.81179672442278,-8.37323013850045));
#31324=CARTESIAN_POINT('Ctrl Pts',(-5.43641663920042,9.09800440456847,-4.59502774450345));
#31325=CARTESIAN_POINT('Ctrl Pts',(-5.37716807645559,10.188354941148,0.292211757959466));
#31326=CARTESIAN_POINT('Ctrl Pts',(-5.31791951371075,8.81968578682977,5.10892422530387));
#31327=CARTESIAN_POINT('Ctrl Pts',(-5.25867095096592,5.32233333254584,8.69256763077374));
#31328=CARTESIAN_POINT('Ctrl Pts',(-5.19942238822108,0.5404042668412,10.1782084546684));
#31329=CARTESIAN_POINT('Ctrl Pts',(-5.14017382547625,-4.37195456312701,
9.2072785021556));
#31330=CARTESIAN_POINT('Ctrl Pts',(-5.08092526273141,-8.2291163155945,6.01411745667809));
#31331=CARTESIAN_POINT('Ctrl Pts',(-5.02167669998658,-10.1001322009791,
1.36941361211582));
#31332=CARTESIAN_POINT('Ctrl Pts',(-4.96242813724175,-9.53342147531196,
-3.60580630266854));
#31333=CARTESIAN_POINT('Ctrl Pts',(-4.9031795744969,-6.66576312219815,-7.71074355150312));
#31334=CARTESIAN_POINT('Ctrl Pts',(-4.84393101175208,-2.18928343658979,
-9.95464726409617));
#31335=CARTESIAN_POINT('Ctrl Pts',(-4.78468244900724,2.815592747828,-9.79593801515108));
#31336=CARTESIAN_POINT('Ctrl Pts',(-4.72543388626241,7.14090897890188,-7.27292122006985));
#31337=CARTESIAN_POINT('Ctrl Pts',(-4.66618532351757,9.74272461626274,-2.99454189651309));
#31338=CARTESIAN_POINT('Ctrl Pts',(-4.60693676077273,9.99307607586648,2.00658781523482));
#31339=CARTESIAN_POINT('Ctrl Pts',(-4.5476881980279,7.83153955304924,6.52341569634566));
#31340=CARTESIAN_POINT('Ctrl Pts',(-4.48843963528306,3.7798146649627,9.46577863764184));
#31341=CARTESIAN_POINT('Ctrl Pts',(-4.42919107253823,-1.18419083591923,
10.1235199502164));
#31342=CARTESIAN_POINT('Ctrl Pts',(-4.36994250979339,-5.8623848785111,8.33788988020998));
#31343=CARTESIAN_POINT('Ctrl Pts',(-4.31069394704856,-9.12565767668712,
4.53986080031373));
#31344=CARTESIAN_POINT('Ctrl Pts',(-4.25144538430373,-10.1863990506059,
-0.353890519962989));
#31345=CARTESIAN_POINT('Ctrl Pts',(-4.19219682155889,-8.78859279937101,
-5.16222827131344));
#31346=CARTESIAN_POINT('Ctrl Pts',(-4.13294825881405,-5.26960772449185,
-8.7246317141917));
#31347=CARTESIAN_POINT('Ctrl Pts',(-4.07369969606922,-0.478771675369725,
-10.1812937194233));
#31348=CARTESIAN_POINT('Ctrl Pts',(-4.01445113332438,4.42761874773907,-9.18064030136098));
#31349=CARTESIAN_POINT('Ctrl Pts',(-3.95520257057955,8.26537721334642,-5.96418507756067));
#31350=CARTESIAN_POINT('Ctrl Pts',(-3.89595400783471,10.1082380298515,-1.30823852953812));
#31351=CARTESIAN_POINT('Ctrl Pts',(-3.83670544508988,9.51141584559089,3.66345912090558));
#31352=CARTESIAN_POINT('Ctrl Pts',(-3.77745688234504,6.61895722269747,7.75095925691813));
#31353=CARTESIAN_POINT('Ctrl Pts',(-3.71820831960021,2.12897414783507,9.96771955846239));
#31354=CARTESIAN_POINT('Ctrl Pts',(-3.65895975685538,-2.8748494224929,9.7787118229497));
#31355=CARTESIAN_POINT('Ctrl Pts',(-3.59971119411054,-7.18481109076589,
7.22955418461685));
#31356=CARTESIAN_POINT('Ctrl Pts',(-3.5404626313657,-9.76067613111137,2.93550090816825));
#31357=CARTESIAN_POINT('Ctrl Pts',(-3.48121406862087,-9.98074428947528,
-2.06705286492883));
#31358=CARTESIAN_POINT('Ctrl Pts',(-3.42196550587603,-7.7919008149599,-6.57071121022154));
#31359=CARTESIAN_POINT('Ctrl Pts',(-3.3627169431312,-3.72243601892731,-9.48848956385033));
#31360=CARTESIAN_POINT('Ctrl Pts',(-3.30346838038636,1.2454607145008,-10.1161648724672));
#31361=CARTESIAN_POINT('Ctrl Pts',(-3.24421981764153,5.91275814226201,-8.3022439899956));
#31362=CARTESIAN_POINT('Ctrl Pts',(-3.1849712548967,9.15297644063244,-4.48452744394893));
#31363=CARTESIAN_POINT('Ctrl Pts',(-3.12572269215187,10.1840697695796,0.415556309830607));
#31364=CARTESIAN_POINT('Ctrl Pts',(-3.06647412940702,8.75717765911764,5.21534309177781));
#31365=CARTESIAN_POINT('Ctrl Pts',(-3.0072255666622,5.21668895481417,8.75637598935904));
#31366=CARTESIAN_POINT('Ctrl Pts',(-2.94797700391735,0.417121534145209,
10.1840057808338));
#31367=CARTESIAN_POINT('Ctrl Pts',(-2.88872844117253,-4.48312063449688,
9.15366557696162));
#31368=CARTESIAN_POINT('Ctrl Pts',(-2.82947987842769,-8.30133513718334,
5.91403407653938));
#31369=CARTESIAN_POINT('Ctrl Pts',(-2.77023131568285,-10.1159733332934,
1.24701549244614));
#31370=CARTESIAN_POINT('Ctrl Pts',(-2.71098275293802,-9.4890615674268,-3.72097765216174));
#31371=CARTESIAN_POINT('Ctrl Pts',(-2.65173419019319,-6.57190870010391,
-7.79089084481372));
#31372=CARTESIAN_POINT('Ctrl Pts',(-2.59248562744835,-2.0685868198553,-9.98042647821348));
#31373=CARTESIAN_POINT('Ctrl Pts',(-2.53323706470351,2.93400071728676,-9.76112718436066));
#31374=CARTESIAN_POINT('Ctrl Pts',(-2.47398850195868,7.22844983771763,-7.18592214415825));
#31375=CARTESIAN_POINT('Ctrl Pts',(-2.41473993921385,9.77826986068487,-2.87635231672436));
#31376=CARTESIAN_POINT('Ctrl Pts',(-2.35549137646901,9.96804665103716,2.1274421451712));
#31377=CARTESIAN_POINT('Ctrl Pts',(-2.29624281372417,7.75197645860605,6.61776586950019));
#31378=CARTESIAN_POINT('Ctrl Pts',(-2.23699425097934,3.6649209240663,9.51085268199676));
#31379=CARTESIAN_POINT('Ctrl Pts',(-2.1777456882345,-1.30668493973852,10.1084389787229));
#31380=CARTESIAN_POINT('Ctrl Pts',(-2.11849712548967,-5.96291466920391,
8.26629377448541));
#31381=CARTESIAN_POINT('Ctrl Pts',(-2.05924856274484,-9.17995969501367,
4.42902970369678));
#31382=CARTESIAN_POINT('Ctrl Pts',(-2.,-10.1813671834506,-0.477206867154204));
#31383=CARTESIAN_POINT('Ctrl Pts',(-1.94075143725517,-8.72544151761641,
-5.26826673973136));
#31384=CARTESIAN_POINT('Ctrl Pts',(-1.88150287451033,-5.163578963292,-8.78779929266436));
#31385=CARTESIAN_POINT('Ctrl Pts',(-1.8222543117655,-0.355456103002113,
-10.1863445394873));
#31386=CARTESIAN_POINT('Ctrl Pts',(-1.76300574902066,4.53845818893508,-9.1263553177373));
#31387=CARTESIAN_POINT('Ctrl Pts',(-1.70375718627583,8.33698876903922,-5.86366629193867));
#31388=CARTESIAN_POINT('Ctrl Pts',(-1.64450862353099,10.1233378277612,-1.18574674501868));
#31389=CARTESIAN_POINT('Ctrl Pts',(-1.58526006078616,9.46635946023347,3.77835978804986));
#31390=CARTESIAN_POINT('Ctrl Pts',(-1.52601149804132,6.52461927901817,7.83053685146607));
#31391=CARTESIAN_POINT('Ctrl Pts',(-1.46676293529649,2.00812366619552,9.99276755756728));
#31392=CARTESIAN_POINT('Ctrl Pts',(-1.40751437255165,-2.99304446397231,
9.74318474396275));
#31393=CARTESIAN_POINT('Ctrl Pts',(-1.34826580980682,-7.27182362014442,
7.14202669806083));
#31394=CARTESIAN_POINT('Ctrl Pts',(-1.28901724706198,-9.7955051600712,2.81709829031974));
#31395=CARTESIAN_POINT('Ctrl Pts',(-1.22976868431715,-9.95498362599407,
-2.1877534423453));
#31396=CARTESIAN_POINT('Ctrl Pts',(-1.17052012157231,-7.71176794744644,
-6.66457794935592));
#31397=CARTESIAN_POINT('Ctrl Pts',(-1.11127155882748,-3.60727148864087,
-9.53286717234345));
#31398=CARTESIAN_POINT('Ctrl Pts',(-1.05202299608264,1.36786126741004,-10.1003425521822));
#31399=CARTESIAN_POINT('Ctrl Pts',(-0.992774433337809,6.01285262080975,
-8.23004055146306));
#31400=CARTESIAN_POINT('Ctrl Pts',(-0.933525870592972,9.20660645073839,
-4.3733696138704));
#31401=CARTESIAN_POINT('Ctrl Pts',(-0.874277307848139,10.1782913912843,
0.538839932083674));
#31402=CARTESIAN_POINT('Ctrl Pts',(-0.815028745103303,8.69338553818084,
5.32099727521684));
#31403=CARTESIAN_POINT('Ctrl Pts',(-0.755780182358468,5.11027969671351,
8.81890047226012));
#31404=CARTESIAN_POINT('Ctrl Pts',(-0.696531619613633,0.293777642336413,
10.1883099096576));
#31405=CARTESIAN_POINT('Ctrl Pts',(-0.637283056868798,-4.59362938261378,
9.09871052476142));
#31406=CARTESIAN_POINT('Ctrl Pts',(-0.578034494123964,-8.37233680199861,
5.81308357004031));
#31407=CARTESIAN_POINT('Ctrl Pts',(-0.518785931379129,-10.1303312433104,
1.12443453308871));
#31408=CARTESIAN_POINT('Ctrl Pts',(-0.459537368634294,-9.44331035616146,
-3.83560342514168));
#31409=CARTESIAN_POINT('Ctrl Pts',(-0.40028880588946,-6.47709069289636,
-7.86989582369838));
#31410=CARTESIAN_POINT('Ctrl Pts',(-0.341040243144624,-1.94758690313188,
-10.0047423439996));
#31411=CARTESIAN_POINT('Ctrl Pts',(-0.281791680399788,3.05197849816094,
-9.72488515974416));
#31412=CARTESIAN_POINT('Ctrl Pts',(-0.222543117654954,7.31493084832684,
-7.09786945477928));
#31413=CARTESIAN_POINT('Ctrl Pts',(-0.163294554910118,9.81238139714809,
-2.75774100205266));
#31414=CARTESIAN_POINT('Ctrl Pts',(-0.104045992165285,9.94155569385488,
2.24798454780788));
#31415=CARTESIAN_POINT('Ctrl Pts',(-0.04479742942045,7.67127675405556,6.71114572977224));
#31416=CARTESIAN_POINT('Ctrl Pts',(0.0144511333243838,3.5494898283465,9.5545322358145));
#31417=CARTESIAN_POINT('Ctrl Pts',(0.0736996960692201,-1.42898745989484,
10.0918758744076));
#31418=CARTESIAN_POINT('Ctrl Pts',(0.132948258814054,-6.06257015720878,
8.1934856791998));
#31419=CARTESIAN_POINT('Ctrl Pts',(0.192196821558891,-9.23291574911109,
4.31754915801126));
#31420=CARTESIAN_POINT('Ctrl Pts',(0.251445384303725,-10.174842470955,-0.600453135899833));
#31421=CARTESIAN_POINT('Ctrl Pts',(0.31069394704856,-8.66101096317135,-5.37353297677851));
#31422=CARTESIAN_POINT('Ctrl Pts',(0.369942509793394,-5.05679297882943,
-8.84967797993003));
#31423=CARTESIAN_POINT('Ctrl Pts',(0.429191072538229,-0.232088663954392,
-10.1899026073391));
#31424=CARTESIAN_POINT('Ctrl Pts',(0.488439635283065,4.64863267764692,-9.07073068997722));
#31425=CARTESIAN_POINT('Ctrl Pts',(0.547688198027898,8.40737700504827,-5.76229070223548));
#31426=CARTESIAN_POINT('Ctrl Pts',(0.606936760772733,10.136955129309,-1.06307543340285));
#31427=CARTESIAN_POINT('Ctrl Pts',(0.666185323517568,9.41991161391276,3.89269551710708));
#31428=CARTESIAN_POINT('Ctrl Pts',(0.725433886262404,6.4293314146994,7.90898745576797));
#31429=CARTESIAN_POINT('Ctrl Pts',(0.784682449007238,1.88696575250372,10.0163095859433));
#31430=CARTESIAN_POINT('Ctrl Pts',(0.843931011752074,-3.11077554156509,
9.7063079455285));
#31431=CARTESIAN_POINT('Ctrl Pts',(0.903179574496908,-7.35781867960586,
7.05329934218052));
#31432=CARTESIAN_POINT('Ctrl Pts',(0.962428137241742,-9.82880151332763,
2.69858197941995));
#31433=CARTESIAN_POINT('Ctrl Pts',(1.02167669998658,-9.92797204235483,-2.30875500923572));
#31434=CARTESIAN_POINT('Ctrl Pts',(1.06117574181647,-8.39592381863737,-5.27349178069045));
#31435=CARTESIAN_POINT('Ctrl Pts',(1.08092526273141,-7.32294389040366,-6.48509627723013));
#31436=CARTESIAN_POINT('Ctrl Pts',(-8.24277578819424,-2.49464822519319,
9.31322804590548));
#31437=CARTESIAN_POINT('Ctrl Pts',(-8.22302626727929,-4.03555160320565,
8.90048051538163));
#31438=CARTESIAN_POINT('Ctrl Pts',(-8.1835272254494,-6.90705648423663,7.29598283929145));
#31439=CARTESIAN_POINT('Ctrl Pts',(-8.12427866270457,-9.54800791581985,
3.12526040329305));
#31440=CARTESIAN_POINT('Ctrl Pts',(-8.06503009995973,-9.88413498448718,
-1.79846037205486));
#31441=CARTESIAN_POINT('Ctrl Pts',(-8.0057815372149,-7.83484886432444,-6.28875651147761));
#31442=CARTESIAN_POINT('Ctrl Pts',(-7.94653297447006,-3.89448213374026,
-9.26089341959434));
#31443=CARTESIAN_POINT('Ctrl Pts',(-7.88728441172523,0.985792474450397,
-9.99802991214653));
#31444=CARTESIAN_POINT('Ctrl Pts',(-7.82803584898039,5.62816531107497,-8.32199426913325));
#31445=CARTESIAN_POINT('Ctrl Pts',(-7.76878728623556,8.91213419563631,-4.63744196065562));
#31446=CARTESIAN_POINT('Ctrl Pts',(-7.70953872349072,10.0451135359474,0.166408123840141));
#31447=CARTESIAN_POINT('Ctrl Pts',(-7.65029016074589,8.75364186156157,4.93008232444777));
#31448=CARTESIAN_POINT('Ctrl Pts',(-7.59104159800104,5.3494287834111,8.50385838389115));
#31449=CARTESIAN_POINT('Ctrl Pts',(-7.53179303525623,0.654098511964837,
10.0251746541477));
#31450=CARTESIAN_POINT('Ctrl Pts',(-7.47254447251138,-4.19910181776543,
9.12685746959272));
#31451=CARTESIAN_POINT('Ctrl Pts',(-7.41329590976655,-8.03882435261888,
6.02571839834814));
#31452=CARTESIAN_POINT('Ctrl Pts',(-7.35404734702171,-9.93832898063206,
1.47023703073982));
#31453=CARTESIAN_POINT('Ctrl Pts',(-7.29479878427688,-9.43915922855823,
-3.44009497269169));
#31454=CARTESIAN_POINT('Ctrl Pts',(-7.23555022153204,-6.66179256465216,
-7.52013959619327));
#31455=CARTESIAN_POINT('Ctrl Pts',(-7.17630165878721,-2.27656290383574,
-9.78515413849957));
#31456=CARTESIAN_POINT('Ctrl Pts',(-7.11705309604237,2.65812868048924,-9.68846385403776));
#31457=CARTESIAN_POINT('Ctrl Pts',(-7.05780453329754,6.9512651900885,-7.25340556462755));
#31458=CARTESIAN_POINT('Ctrl Pts',(-6.99855597055269,9.5666727579438,-3.0676949566889));
#31459=CARTESIAN_POINT('Ctrl Pts',(-6.93930740780788,9.87310730343358,1.85842195835291));
#31460=CARTESIAN_POINT('Ctrl Pts',(-6.88005884506304,7.7966090395667,6.33599775053658));
#31461=CARTESIAN_POINT('Ctrl Pts',(-6.8208102823182,3.83835309599371,9.28434303076916));
#31462=CARTESIAN_POINT('Ctrl Pts',(-6.76156171957337,-1.04631205655837,
9.99185723914637));
#31463=CARTESIAN_POINT('Ctrl Pts',(-6.70231315682853,-5.67844360934779,
8.28777763821964));
#31464=CARTESIAN_POINT('Ctrl Pts',(-6.64306459408369,-8.94004923030717,
4.5833939134041));
#31465=CARTESIAN_POINT('Ctrl Pts',(-6.58381603133887,-10.043921122745,-0.227219026059686));
#31466=CARTESIAN_POINT('Ctrl Pts',(-6.52456746859402,-8.7236332801272,-4.98299131039099));
#31467=CARTESIAN_POINT('Ctrl Pts',(-6.46531890584919,-5.29784497783292,
-8.53608918630591));
#31468=CARTESIAN_POINT('Ctrl Pts',(-6.40607034310436,-0.593390473281026,
-10.0289514781879));
#31469=CARTESIAN_POINT('Ctrl Pts',(-6.34682178035952,4.25428232967126,-9.1012670472368));
#31470=CARTESIAN_POINT('Ctrl Pts',(-6.28757321761468,8.07515894425764,-5.9769380146219));
#31471=CARTESIAN_POINT('Ctrl Pts',(-6.22832465486986,9.94704821341236,-1.41003966104096));
#31472=CARTESIAN_POINT('Ctrl Pts',(-6.16907609212501,9.4181585968316,3.49718009982154));
#31473=CARTESIAN_POINT('Ctrl Pts',(-6.10982752938019,6.61614072987225,7.56033477090688));
#31474=CARTESIAN_POINT('Ctrl Pts',(-6.05057896663535,2.21727818813639,9.79875795405083));
#31475=CARTESIAN_POINT('Ctrl Pts',(-5.99133040389051,-2.71673755117854,
9.67219298213572));
#31476=CARTESIAN_POINT('Ctrl Pts',(-5.93208184114568,-6.99505262321808,
7.21118705928984));
#31477=CARTESIAN_POINT('Ctrl Pts',(-5.87283327840084,-9.58507039518135,
3.00971851259834));
#31478=CARTESIAN_POINT('Ctrl Pts',(-5.81358471565601,-9.8616747675781,-1.9181633882891));
#31479=CARTESIAN_POINT('Ctrl Pts',(-5.75433615291117,-7.75810564005444,
-6.38308521668124));
#31480=CARTESIAN_POINT('Ctrl Pts',(-5.69508759016634,-3.78207185624856,
-9.30741169605342));
#31481=CARTESIAN_POINT('Ctrl Pts',(-5.6358390274215,1.10678732681236,-9.98533934420192));
#31482=CARTESIAN_POINT('Ctrl Pts',(-5.57659046467667,5.7285168460572,-8.25324631585039));
#31483=CARTESIAN_POINT('Ctrl Pts',(-5.51734190193183,8.96763496184554,-4.52918350221593));
#31484=CARTESIAN_POINT('Ctrl Pts',(-5.458093339187,10.0423613697144,0.288024522786977));
#31485=CARTESIAN_POINT('Ctrl Pts',(-5.39884477644216,8.69330449815474,5.03571612663202));
#31486=CARTESIAN_POINT('Ctrl Pts',(-5.33959621369733,5.24606719772168,8.56800787596791));
#31487=CARTESIAN_POINT('Ctrl Pts',(-5.2803476509525,0.532660568335423,10.0323602768541));
#31488=CARTESIAN_POINT('Ctrl Pts',(-5.22109908820766,-4.30930683790513,
9.07534322119243));
#31489=CARTESIAN_POINT('Ctrl Pts',(-5.16185052546282,-8.11119756545325,
5.92793843252815));
#31490=CARTESIAN_POINT('Ctrl Pts',(-5.102601962718,-9.95540281331162,1.34979066168298));
#31491=CARTESIAN_POINT('Ctrl Pts',(-5.04335339997315,-9.39681274336244,
-3.55413706430132));
#31492=CARTESIAN_POINT('Ctrl Pts',(-4.98410483722832,-6.57024637095018,
-7.60025280044521));
#31493=CARTESIAN_POINT('Ctrl Pts',(-4.92485627448348,-2.1579121985799,-9.8120025962532));
#31494=CARTESIAN_POINT('Ctrl Pts',(-4.86560771173865,2.77524683886309,-9.65556756431436));
#31495=CARTESIAN_POINT('Ctrl Pts',(-4.80635914899381,7.03858364658536,-7.16870422431282));
#31496=CARTESIAN_POINT('Ctrl Pts',(-4.74711058624898,9.60311668441919,-2.95163174381379));
#31497=CARTESIAN_POINT('Ctrl Pts',(-4.68786202350415,9.8498807441029,1.97783450587003));
#31498=CARTESIAN_POINT('Ctrl Pts',(-4.62861346075931,7.71931786114931,6.42993870609979));
#31499=CARTESIAN_POINT('Ctrl Pts',(-4.56936489801447,3.72565198163625,9.33013919067606));
#31500=CARTESIAN_POINT('Ctrl Pts',(-4.51011633526964,-1.1672220268825,9.97845542885368));
#31501=CARTESIAN_POINT('Ctrl Pts',(-4.45086777252481,-5.77838009947901,
8.21841246419309));
#31502=CARTESIAN_POINT('Ctrl Pts',(-4.39161920977997,-8.99489197765177,
4.47480707025844));
#31503=CARTESIAN_POINT('Ctrl Pts',(-4.33237064703514,-10.0404335060174,
-0.348819461759353));
#31504=CARTESIAN_POINT('Ctrl Pts',(-4.2731220842903,-8.66265705625382,-5.08825635472459));
#31505=CARTESIAN_POINT('Ctrl Pts',(-4.21387352154547,-5.19409711888415,
-8.5996124985524));
#31506=CARTESIAN_POINT('Ctrl Pts',(-4.15462495880063,-0.471911138296548,
-10.0354013314471));
#31507=CARTESIAN_POINT('Ctrl Pts',(-4.0953763960558,4.3641733851008,-9.04908673129157));
#31508=CARTESIAN_POINT('Ctrl Pts',(-4.03612783331096,8.14693886431048,-5.87872155717949));
#31509=CARTESIAN_POINT('Ctrl Pts',(-3.97687927056613,9.96339249007565,-1.28949218468484));
#31510=CARTESIAN_POINT('Ctrl Pts',(-3.91763070782129,9.37512244231739,3.61096374908634));
#31511=CARTESIAN_POINT('Ctrl Pts',(-3.85838214507646,6.52411117446994,7.63989223672795));
#31512=CARTESIAN_POINT('Ctrl Pts',(-3.79913358233162,2.09846710905133,9.82488757176839));
#31513=CARTESIAN_POINT('Ctrl Pts',(-3.73988501958679,-2.83365439768783,
9.6385882140552));
#31514=CARTESIAN_POINT('Ctrl Pts',(-3.68063645684195,-7.08185666512257,
7.12595861483339));
#31515=CARTESIAN_POINT('Ctrl Pts',(-3.62138789409712,-9.62081096384753,
2.89343678064173));
#31516=CARTESIAN_POINT('Ctrl Pts',(-3.56213933135228,-9.83772566548719,
-2.03743312436855));
#31517=CARTESIAN_POINT('Ctrl Pts',(-3.50289076860745,-7.68024712456503,
-6.4765565010482));
#31518=CARTESIAN_POINT('Ctrl Pts',(-3.44364220586261,-3.6690955403147,-9.35252468169435));
#31519=CARTESIAN_POINT('Ctrl Pts',(-3.38439364311778,1.22761394150943,-9.97120574535853));
#31520=CARTESIAN_POINT('Ctrl Pts',(-3.32514508037294,5.82803154182476,-8.18327736015069));
#31521=CARTESIAN_POINT('Ctrl Pts',(-3.26589651762811,9.02181927860445,-4.42026661072162));
#31522=CARTESIAN_POINT('Ctrl Pts',(-3.20664795488328,10.0381376023182,0.409601614479463));
#31523=CARTESIAN_POINT('Ctrl Pts',(-3.14739939213844,8.6316920778322,5.14061006877085));
#31524=CARTESIAN_POINT('Ctrl Pts',(-3.08815082939361,5.14193664632369,8.63090189556414));
#31525=CARTESIAN_POINT('Ctrl Pts',(-3.02890226664877,0.411144409983018,
10.0380745304963));
#31526=CARTESIAN_POINT('Ctrl Pts',(-2.96965370390394,-4.41887996008199,
9.02249853998576));
#31527=CARTESIAN_POINT('Ctrl Pts',(-2.9104051411591,-8.18238153070373,5.82928919265959));
#31528=CARTESIAN_POINT('Ctrl Pts',(-2.85115657841427,-9.97101695083666,
1.22914644033452));
#31529=CARTESIAN_POINT('Ctrl Pts',(-2.79190801566943,-9.35308848877147,
-3.66765807114975));
#31530=CARTESIAN_POINT('Ctrl Pts',(-2.7326594529246,-6.47773683155344,-7.6792516267404));
#31531=CARTESIAN_POINT('Ctrl Pts',(-2.67341089017976,-2.03894509855726,
-9.83741240828749));
#31532=CARTESIAN_POINT('Ctrl Pts',(-2.61416232743493,2.89195808667764,-9.62125555374968));
#31533=CARTESIAN_POINT('Ctrl Pts',(-2.55491376469009,7.12487009262311,-7.08295179772558));
#31534=CARTESIAN_POINT('Ctrl Pts',(-2.49566520194526,9.63815258486866,-2.83513575626437));
#31535=CARTESIAN_POINT('Ctrl Pts',(-2.43641663920042,9.8252099772849,2.09695705915036));
#31536=CARTESIAN_POINT('Ctrl Pts',(-2.37716807645559,7.64089486247027,6.52293689271442));
#31537=CARTESIAN_POINT('Ctrl Pts',(-2.31791951371075,3.61240460540479,9.37456734855053));
#31538=CARTESIAN_POINT('Ctrl Pts',(-2.25867095096591,-1.28796085698004,
9.9635905594593));
#31539=CARTESIAN_POINT('Ctrl Pts',(-2.19942238822108,-5.87746935308181,
8.14784229162806));
#31540=CARTESIAN_POINT('Ctrl Pts',(-2.14017382547625,-9.04841587766215,
4.36556412282892));
#31541=CARTESIAN_POINT('Ctrl Pts',(-2.08092526273141,-10.035473742775,-0.470368752929598));
#31542=CARTESIAN_POINT('Ctrl Pts',(-2.02167669998658,-8.60041069793557,
-5.19277534970414));
#31543=CARTESIAN_POINT('Ctrl Pts',(-1.96242813724174,-5.08958769202351,
-8.66187492006564));
#31544=CARTESIAN_POINT('Ctrl Pts',(-1.90317957449691,-0.350362610847111,
-10.0403797760134));
#31545=CARTESIAN_POINT('Ctrl Pts',(-1.84393101175207,4.47342455753611,-8.99557962188608));
#31546=CARTESIAN_POINT('Ctrl Pts',(-1.78468244900724,8.21752426545409,-5.7796431509508));
#31547=CARTESIAN_POINT('Ctrl Pts',(-1.7254338862624,9.97827591611403,-1.16875564065287));
#31548=CARTESIAN_POINT('Ctrl Pts',(-1.66618532351757,9.3307116903966,3.72421795231635));
#31549=CARTESIAN_POINT('Ctrl Pts',(-1.60693676077273,6.43112504208883,7.71832952773314));
#31550=CARTESIAN_POINT('Ctrl Pts',(-1.5476881980279,1.97934834892384,9.84957664670273));
#31551=CARTESIAN_POINT('Ctrl Pts',(-1.48843963528306,-2.9501557686649,9.60357021874013));
#31552=CARTESIAN_POINT('Ctrl Pts',(-1.42919107253823,-7.16762235239588,
7.03968534943816));
#31553=CARTESIAN_POINT('Ctrl Pts',(-1.36994250979339,-9.65514091181178,
2.77673080775176));
#31554=CARTESIAN_POINT('Ctrl Pts',(-1.31069394704856,-9.81233413826848,
-2.15640412831874));
#31555=CARTESIAN_POINT('Ctrl Pts',(-1.25144538430372,-7.60126251735319,
-6.56907818098861));
#31556=CARTESIAN_POINT('Ctrl Pts',(-1.19219682155889,-3.5555812549575,-9.39626638325325));
#31557=CARTESIAN_POINT('Ctrl Pts',(-1.13294825881405,1.34826056123045,-9.95561015029659));
#31558=CARTESIAN_POINT('Ctrl Pts',(-1.07369969606922,5.9266917210682,-8.11210855752574));
#31559=CARTESIAN_POINT('Ctrl Pts',(-1.01445113332438,9.07468079990562,-4.31070161174287));
#31560=CARTESIAN_POINT('Ctrl Pts',(-0.955202570579551,10.0324420250335,
0.531118649642064));
#31561=CARTESIAN_POINT('Ctrl Pts',(-0.895954007834716,8.5688140632078,5.24475028536576));
#31562=CARTESIAN_POINT('Ctrl Pts',(-0.836705445089879,5.03705217487539,
8.6925304367147));
#31563=CARTESIAN_POINT('Ctrl Pts',(-0.777456882345046,0.289567968894557,
10.0423169835008));
#31564=CARTESIAN_POINT('Ctrl Pts',(-0.71820831960021,-4.52780517808973,
8.96833096372111));
#31565=CARTESIAN_POINT('Ctrl Pts',(-0.658959756855376,-8.25236578037355,
5.72978525187863));
#31566=CARTESIAN_POINT('Ctrl Pts',(-0.59971119411054,-9.9851691198313,1.10832199929135));
#31567=CARTESIAN_POINT('Ctrl Pts',(-0.540462631365706,-9.30799286741916,
-3.78064131929891));
#31568=CARTESIAN_POINT('Ctrl Pts',(-0.481214068620872,-6.38427751469271,
-7.75712450735258));
#31569=CARTESIAN_POINT('Ctrl Pts',(-0.421965505876037,-1.91967904466917,
-9.86137984097431));
#31570=CARTESIAN_POINT('Ctrl Pts',(-0.3627169431312,3.00824531027549,-9.58553285758615));
#31571=CARTESIAN_POINT('Ctrl Pts',(-0.303468380386366,7.21011187750129,
-6.99616085537751));
#31572=CARTESIAN_POINT('Ctrl Pts',(-0.24421981764153,9.67177532161258,-2.71822407706291));
#31573=CARTESIAN_POINT('Ctrl Pts',(-0.184971254896697,9.7990986210757,2.21577215487913));
#31574=CARTESIAN_POINT('Ctrl Pts',(-0.125722692151862,7.56135154068707,
6.61497867050113));
#31575=CARTESIAN_POINT('Ctrl Pts',(-0.0664741294070281,3.49862757435156,
9.41762099817694));
#31576=CARTESIAN_POINT('Ctrl Pts',(-0.00722556666219214,-1.40851084870404,
9.94726479539839));
#31577=CARTESIAN_POINT('Ctrl Pts',(0.0520229960826427,-5.97569683227752,
8.07607749665164));
#31578=CARTESIAN_POINT('Ctrl Pts',(0.111271558827478,-9.10061310037694,
4.25568103258189));
#31579=CARTESIAN_POINT('Ctrl Pts',(0.170520121572313,-10.029042525852,-0.591848969840164));
#31580=CARTESIAN_POINT('Ctrl Pts',(0.229768684317147,-8.53690339820701,
-5.29653317896745));
#31581=CARTESIAN_POINT('Ctrl Pts',(0.289017247061983,-4.98433189249667,
-8.72286691948016));
#31582=CARTESIAN_POINT('Ctrl Pts',(0.348265809806816,-0.228762959938813,
-10.0438868586929));
#31583=CARTESIAN_POINT('Ctrl Pts',(0.407514372551653,4.58202030589382,-8.94075206471425));
#31584=CARTESIAN_POINT('Ctrl Pts',(0.466762935296486,8.28690387641807,-5.67972021817628));
#31585=CARTESIAN_POINT('Ctrl Pts',(0.526011498041321,9.991698089155,-1.0478421420499));
#31586=CARTESIAN_POINT('Ctrl Pts',(0.585260060786157,9.28492941638948,3.83691531271406));
#31587=CARTESIAN_POINT('Ctrl Pts',(0.644508623530991,6.3372026009131,7.79565597764807));
#31588=CARTESIAN_POINT('Ctrl Pts',(0.703757186275827,1.85992656207777,9.87278133064767));
#31589=CARTESIAN_POINT('Ctrl Pts',(0.76300574902066,-3.06619982410485,9.56722184472157));
#31590=CARTESIAN_POINT('Ctrl Pts',(0.822254311765497,-7.25238514954131,
6.95222940819188));
#31591=CARTESIAN_POINT('Ctrl Pts',(0.881502874510329,-9.6879601464798,2.65991277096996));
#31592=CARTESIAN_POINT('Ctrl Pts',(0.940751437255167,-9.7857096158956,-2.27567180872784));
#31593=CARTESIAN_POINT('Ctrl Pts',(0.980250479085055,-8.27561480792394,
-5.19792551867508));
#31594=CARTESIAN_POINT('Ctrl Pts',(1.,-7.218010097054,-6.39216838336776));
#31595=CARTESIAN_POINT('Ctrl Pts',(1.,-7.218010097054,-6.39216838336776));
#31596=CARTESIAN_POINT('Ctrl Pts',(1.,-7.38033772502723,-6.21660074016268));
#31597=CARTESIAN_POINT('Ctrl Pts',(0.999999999999999,-7.53570865858123,
-6.03520929800804));
#31598=CARTESIAN_POINT('Ctrl Pts',(0.999999999999999,-7.68398068614723,
-5.84850759966542));
#31599=CARTESIAN_POINT('Ctrl Pts',(1.,-7.83425301467726,-5.65928715524971));
#31600=CARTESIAN_POINT('Ctrl Pts',(1.,-7.97723397958538,-5.46461174998116));
#31601=CARTESIAN_POINT('Ctrl Pts',(1.,-8.11274192803781,-5.26497371679585));
#31602=CARTESIAN_POINT('Ctrl Pts',(1.,-8.24926802235148,-5.06383569309665));
#31603=CARTESIAN_POINT('Ctrl Pts',(0.999999999999998,-8.37820875008256,
-4.85765966198851));
#31604=CARTESIAN_POINT('Ctrl Pts',(0.999999999999998,-8.49933886135329,
-4.64691404211075));
#31605=CARTESIAN_POINT('Ctrl Pts',(0.999999999999997,-8.62014279896438,
-4.43673590846219));
#31606=CARTESIAN_POINT('Ctrl Pts',(1.,-8.73317843953205,-4.22201218564418));
#31607=CARTESIAN_POINT('Ctrl Pts',(1.,-8.83817822275541,-4.00318110377646));
#31608=CARTESIAN_POINT('Ctrl Pts',(1.,-8.90711959723496,-3.85949970654237));
#31609=CARTESIAN_POINT('Ctrl Pts',(1.,-8.97259576417475,-3.71404708405175));
#31610=CARTESIAN_POINT('Ctrl Pts',(1.,-9.03451959595587,-3.56694287159514));
#31611=CARTESIAN_POINT('Ctrl Pts',(1.,-9.06021095437682,-3.50591132786227));
#31612=CARTESIAN_POINT('Ctrl Pts',(1.,-9.08529073461529,-3.44459546100671));
#31613=CARTESIAN_POINT('Ctrl Pts',(1.,-9.10975222670468,-3.38300368933708));
#31614=CARTESIAN_POINT('Ctrl Pts',(1.,-9.12543439611011,-3.34351743912086));
#31615=CARTESIAN_POINT('Ctrl Pts',(0.999999999999998,-9.1408624405508,-3.30391778949324));
#31616=CARTESIAN_POINT('Ctrl Pts',(0.999999999999998,-9.15603452786866,
-3.26420694634604));
#31617=CARTESIAN_POINT('Ctrl Pts',(0.999999999999998,-9.16539765652395,
-3.23970025022654));
#31618=CARTESIAN_POINT('Ctrl Pts',(1.,-9.17466411167333,-3.21514903349331));
#31619=CARTESIAN_POINT('Ctrl Pts',(1.,-9.18383080790029,-3.19056092275229));
#31620=CARTESIAN_POINT('Ctrl Pts',(1.,-9.26956815148778,-2.96058501359442));
#31621=CARTESIAN_POINT('Ctrl Pts',(1.,-9.34642884496221,-2.72779994416276));
#31622=CARTESIAN_POINT('Ctrl Pts',(1.,-9.41421857063004,-2.492691400286));
#31623=CARTESIAN_POINT('Ctrl Pts',(1.,-9.4415819795859,-2.39778953762557));
#31624=CARTESIAN_POINT('Ctrl Pts',(1.,-9.46746693113579,-2.30250875679181));
#31625=CARTESIAN_POINT('Ctrl Pts',(1.,-9.49185860296011,-2.20687973654423));
#31626=CARTESIAN_POINT('Ctrl Pts',(1.,-9.55185343242315,-1.97166638984157));
#31627=CARTESIAN_POINT('Ctrl Pts',(1.,-9.60281768869445,-1.7343475047727));
#31628=CARTESIAN_POINT('Ctrl Pts',(1.,-9.64482604864012,-1.49544925869656));
#31629=CARTESIAN_POINT('Ctrl Pts',(1.,-9.6871492900488,-1.25476030645304));
#31630=CARTESIAN_POINT('Ctrl Pts',(1.,-9.72038194639541,-1.01246759088605));
#31631=CARTESIAN_POINT('Ctrl Pts',(1.,-9.74454903488948,-0.769095725160656));
#31632=CARTESIAN_POINT('Ctrl Pts',(1.,-9.76872045220789,-0.525680266511232));
#31633=CARTESIAN_POINT('Ctrl Pts',(1.,-9.78382307936487,-0.28118460779274));
#31634=CARTESIAN_POINT('Ctrl Pts',(1.,-9.78983010083248,-0.0361300070823768));
#31635=CARTESIAN_POINT('Ctrl Pts',(1.,-9.79255545728033,0.0750500743810585));
#31636=CARTESIAN_POINT('Ctrl Pts',(1.,-9.79340787224445,0.186345196742594));
#31637=CARTESIAN_POINT('Ctrl Pts',(1.,-9.79238129738034,0.29770636029337));
#31638=CARTESIAN_POINT('Ctrl Pts',(1.,-9.7918485179152,0.355501405961876));
#31639=CARTESIAN_POINT('Ctrl Pts',(1.,-9.79080959995854,0.413314234074637));
#31640=CARTESIAN_POINT('Ctrl Pts',(1.,-9.78926346177246,0.471137948752055));
#31641=CARTESIAN_POINT('Ctrl Pts',(1.,-9.78827695465579,0.508032132308922));
#31642=CARTESIAN_POINT('Ctrl Pts',(1.,-9.78708370731581,0.544935718081712));
#31643=CARTESIAN_POINT('Ctrl Pts',(1.,-9.78568473007052,0.581816524025753));
#31644=CARTESIAN_POINT('Ctrl Pts',(1.,-9.7763473698279,0.827974474268892));
#31645=CARTESIAN_POINT('Ctrl Pts',(0.999999999999998,-9.75784570194124,
1.07334621400395));
#31646=CARTESIAN_POINT('Ctrl Pts',(0.999999999999998,-9.730258741531,1.3174026125394));
#31647=CARTESIAN_POINT('Ctrl Pts',(0.999999999999998,-9.70256575117013,
1.56239703713871));
#31648=CARTESIAN_POINT('Ctrl Pts',(0.999999999999996,-9.66571752447539,
1.80606665550865));
#31649=CARTESIAN_POINT('Ctrl Pts',(0.999999999999996,-9.61974203609876,
2.04788259603852));
#31650=CARTESIAN_POINT('Ctrl Pts',(0.999999999999996,-9.58407738698297,
2.23546691485976));
#31651=CARTESIAN_POINT('Ctrl Pts',(0.999999999999998,-9.54291928114351,
2.42193598770508));
#31652=CARTESIAN_POINT('Ctrl Pts',(0.999999999999999,-9.4962591980495,2.60704169439268));
#31653=CARTESIAN_POINT('Ctrl Pts',(0.999999999999999,-9.4361780998623,2.84539005129771));
#31654=CARTESIAN_POINT('Ctrl Pts',(1.,-9.36697631765938,3.08147877897739));
#31655=CARTESIAN_POINT('Ctrl Pts',(1.,-9.28891866527466,3.31486192371426));
#31656=CARTESIAN_POINT('Ctrl Pts',(1.,-9.2337641129153,3.47976750930297));
#31657=CARTESIAN_POINT('Ctrl Pts',(0.999999999999998,-9.17418703363605,
3.64332206604504));
#31658=CARTESIAN_POINT('Ctrl Pts',(0.999999999999998,-9.1102663177799,3.8053623967777));
#31659=CARTESIAN_POINT('Ctrl Pts',(0.999999999999998,-9.07823122598397,
3.88657201403772));
#31660=CARTESIAN_POINT('Ctrl Pts',(1.,-9.04510495830855,3.96740121333635));
#31661=CARTESIAN_POINT('Ctrl Pts',(1.,-9.01089637781328,4.04782884761811));
#31662=CARTESIAN_POINT('Ctrl Pts',(1.,-8.98491018784549,4.1089248578251));
#31663=CARTESIAN_POINT('Ctrl Pts',(0.999999999999997,-8.95829943234446,
4.16978913592025));
#31664=CARTESIAN_POINT('Ctrl Pts',(0.999999999999996,-8.93106773262397,
4.23041223277627));
#31665=CARTESIAN_POINT('Ctrl Pts',(0.999999999999996,-8.91985573978134,
4.2553723246921));
#31666=CARTESIAN_POINT('Ctrl Pts',(1.,-8.90854184623664,4.28028401514663));
#31667=CARTESIAN_POINT('Ctrl Pts',(1.,-8.89712824313656,4.30514296030326));
#31668=CARTESIAN_POINT('Ctrl Pts',(1.,-8.79449431220153,4.52868071940972));
#31669=CARTESIAN_POINT('Ctrl Pts',(0.999999999999998,-8.68375800201423,
4.74805239366863));
#31670=CARTESIAN_POINT('Ctrl Pts',(0.999999999999999,-8.56525007473062,
4.96284307910226));
#31671=CARTESIAN_POINT('Ctrl Pts',(0.999999999999999,-8.44538160194408,
5.18009969662868));
#31672=CARTESIAN_POINT('Ctrl Pts',(0.999999999999999,-8.31756182226729,
5.39267013902898));
#31673=CARTESIAN_POINT('Ctrl Pts',(0.999999999999999,-8.18208200192093,
5.60011072880211));
#31674=CARTESIAN_POINT('Ctrl Pts',(0.999999999999999,-8.04666336029153,
5.80745764448343));
#31675=CARTESIAN_POINT('Ctrl Pts',(1.,-7.90359128193536,6.00967992523946));
#31676=CARTESIAN_POINT('Ctrl Pts',(1.,-7.75311011393737,6.20631136198203));
#31677=CARTESIAN_POINT('Ctrl Pts',(1.,-7.60409271693618,6.40103011158911));
#31678=CARTESIAN_POINT('Ctrl Pts',(1.,-7.44780931337785,6.59026678062805));
#31679=CARTESIAN_POINT('Ctrl Pts',(1.,-7.28445663684239,6.77353773959716));
#31680=CARTESIAN_POINT('Ctrl Pts',(1.,-7.25089458908372,6.81119214972472));
#31681=CARTESIAN_POINT('Ctrl Pts',(1.,-7.2170339997554,6.84859461006606));
#31682=CARTESIAN_POINT('Ctrl Pts',(1.,-7.18287638116905,6.88574073117186));
#31683=CARTESIAN_POINT('Ctrl Pts',(1.,-7.04310063062746,7.03774567683707));
#31684=CARTESIAN_POINT('Ctrl Pts',(1.,-6.89835224551882,7.18545977217479));
#31685=CARTESIAN_POINT('Ctrl Pts',(1.,-6.74886883975424,7.32870626947399));
#31686=CARTESIAN_POINT('Ctrl Pts',(1.,-6.72044540624219,7.35594378972577));
#31687=CARTESIAN_POINT('Ctrl Pts',(1.,-6.69184773627237,7.3830224478866));
#31688=CARTESIAN_POINT('Ctrl Pts',(1.,-6.66309768238747,7.4099222241242));
#31689=CARTESIAN_POINT('Ctrl Pts',(1.,-6.48228040589527,7.57910257755957));
#31690=CARTESIAN_POINT('Ctrl Pts',(1.,-6.29529510224086,7.74135043073779));
#31691=CARTESIAN_POINT('Ctrl Pts',(1.,-6.10262676105486,7.89643853847066));
#31692=CARTESIAN_POINT('Ctrl Pts',(1.,-5.90856004843239,8.05265226330623));
#31693=CARTESIAN_POINT('Ctrl Pts',(1.,-5.70872700746814,8.20160234411627));
#31694=CARTESIAN_POINT('Ctrl Pts',(1.,-5.50358541811632,8.34301973665858));
#31695=CARTESIAN_POINT('Ctrl Pts',(1.,-5.3158480140083,8.47243929636612));
#31696=CARTESIAN_POINT('Ctrl Pts',(0.999999999999999,-5.12366386476961,
8.59554989096275));
#31697=CARTESIAN_POINT('Ctrl Pts',(0.999999999999999,-4.92736180550962,
8.71211419861635));
#31698=CARTESIAN_POINT('Ctrl Pts',(0.999999999999999,-4.89295954817348,
8.73254228441038));
#31699=CARTESIAN_POINT('Ctrl Pts',(1.,-4.85843077260399,8.75276923386899));
#31700=CARTESIAN_POINT('Ctrl Pts',(1.,-4.82377719504876,8.77279366648196));
#31701=CARTESIAN_POINT('Ctrl Pts',(1.,-4.79450813505122,8.78970667693901));
#31702=CARTESIAN_POINT('Ctrl Pts',(0.999999999999996,-4.76515157312949,
8.80647428626319));
#31703=CARTESIAN_POINT('Ctrl Pts',(0.999999999999996,-4.73571877009977,
8.82309006334544));
#31704=CARTESIAN_POINT('Ctrl Pts',(0.999999999999997,-4.51751740444002,
8.94627184957165));
#31705=CARTESIAN_POINT('Ctrl Pts',(1.,-4.29497551340846,9.06120098158676));
#31706=CARTESIAN_POINT('Ctrl Pts',(0.999999999999999,-4.06855850342775,
9.16761502395632));
#31707=CARTESIAN_POINT('Ctrl Pts',(0.999999999999999,-3.84298106373966,
9.27363447552769));
#31708=CARTESIAN_POINT('Ctrl Pts',(1.,-3.61355662653113,9.37120220887847));
#31709=CARTESIAN_POINT('Ctrl Pts',(1.,-3.38071834466137,9.46001497115018));
#31710=CARTESIAN_POINT('Ctrl Pts',(1.,-3.27719789143318,9.4995013362315));
#31711=CARTESIAN_POINT('Ctrl Pts',(0.999999999999997,-3.17300231116554,
9.53725648506412));
#31712=CARTESIAN_POINT('Ctrl Pts',(0.999999999999997,-3.06816838561069,
9.57325070271326));
#31713=CARTESIAN_POINT('Ctrl Pts',(0.999999999999997,-2.91468505697523,
9.62594845591844));
#31714=CARTESIAN_POINT('Ctrl Pts',(0.999999999999999,-2.75983351721763,
9.67487209480759));
#31715=CARTESIAN_POINT('Ctrl Pts',(0.999999999999999,-2.60375578640692,
9.7200109471421));
#31716=CARTESIAN_POINT('Ctrl Pts',(0.16348406216194,-9.64208031777467,-0.000174349252608778));
#31717=CARTESIAN_POINT('Ctrl Pts',(0.165829415298731,-9.64223943100266,
-0.189581381928583));
#31718=CARTESIAN_POINT('Ctrl Pts',(0.168174768435523,-9.63677165214438,
-0.378979236144793));
#31719=CARTESIAN_POINT('Ctrl Pts',(0.170520121572314,-9.62561443366536,
-0.568041337624323));
#31720=CARTESIAN_POINT('Ctrl Pts',(0.19026964248726,-9.53166281663704,-2.16007703954927));
#31721=CARTESIAN_POINT('Ctrl Pts',(0.210019163402205,-9.034283107422,-3.72830510925844));
#31722=CARTESIAN_POINT('Ctrl Pts',(0.229768684317151,-8.19349800186272,
-5.0834747675318));
#31723=CARTESIAN_POINT('Ctrl Pts',(0.249518205232095,-7.35271289630349,
-6.43864442580509));
#31724=CARTESIAN_POINT('Ctrl Pts',(0.26926772614704,-6.16852239440005,-7.58075567264264));
#31725=CARTESIAN_POINT('Ctrl Pts',(0.289017247061984,-4.78383232135538,
-8.37198128593018));
#31726=CARTESIAN_POINT('Ctrl Pts',(0.308766767976929,-3.39914224831071,
-9.16320689921773));
#31727=CARTESIAN_POINT('Ctrl Pts',(0.328516288891873,-1.81395260412477,
-9.60354687895529));
#31728=CARTESIAN_POINT('Ctrl Pts',(0.348265809806818,-0.219560571059729,
-9.63986106982765));
#31729=CARTESIAN_POINT('Ctrl Pts',(0.368015330721763,1.37483146200536,-9.6761752607));
#31730=CARTESIAN_POINT('Ctrl Pts',(0.387764851636707,2.97842588394947,-9.30846366270717));
#31731=CARTESIAN_POINT('Ctrl Pts',(0.407514372551652,4.39770369000897,-8.58110255595442));
#31732=CARTESIAN_POINT('Ctrl Pts',(0.427263893466598,5.81698149606851,-7.85374144920165));
#31733=CARTESIAN_POINT('Ctrl Pts',(0.447013414381543,7.05194268624332,-6.76673083368895));
#31734=CARTESIAN_POINT('Ctrl Pts',(0.466762935296488,7.95355565012021,-5.45124584657818));
#31735=CARTESIAN_POINT('Ctrl Pts',(0.486512456211433,8.85516861399705,-4.13576085946748));
#31736=CARTESIAN_POINT('Ctrl Pts',(0.506261977126377,9.42343335157602,-2.5918015007587));
#31737=CARTESIAN_POINT('Ctrl Pts',(0.526011498041322,9.58977094157126,-1.00569557894368));
#31738=CARTESIAN_POINT('Ctrl Pts',(0.545761018956267,9.7561085315665,0.580410342871385));
#31739=CARTESIAN_POINT('Ctrl Pts',(0.565510539871213,9.52051897397799,2.20866282779273));
#31740=CARTESIAN_POINT('Ctrl Pts',(0.585260060786158,8.91143639260434,3.68257918107574));
#31741=CARTESIAN_POINT('Ctrl Pts',(0.605009581701103,8.30235381123068,5.15649553435874));
#31742=CARTESIAN_POINT('Ctrl Pts',(0.624759102616048,7.31977820607187,6.47607575600343));
#31743=CARTESIAN_POINT('Ctrl Pts',(0.644508623530993,6.08227773035324,7.48205342565903));
#31744=CARTESIAN_POINT('Ctrl Pts',(0.664258144445937,4.84477725463465,8.48803109531461));
#31745=CARTESIAN_POINT('Ctrl Pts',(0.684007665360883,3.35235190835623,9.18040621298113));
#31746=CARTESIAN_POINT('Ctrl Pts',(0.703757186275827,1.78511817085327,9.47566719082672));
#31747=CARTESIAN_POINT('Ctrl Pts',(0.723506707190773,0.217884433350224,
9.77092816867232));
#31748=CARTESIAN_POINT('Ctrl Pts',(0.743256228105716,-1.42415769537726,
9.66907500669695));
#31749=CARTESIAN_POINT('Ctrl Pts',(0.763005749020662,-2.94287631398048,
9.18231635295431));
#31750=CARTESIAN_POINT('Ctrl Pts',(0.782755269935607,-4.46159493258366,
8.69555769921168));
#31751=CARTESIAN_POINT('Ctrl Pts',(0.802504790850553,-5.8569900410625,7.82389355370177));
#31752=CARTESIAN_POINT('Ctrl Pts',(0.822254311765498,-6.96061676145832,
6.67267537474318));
#31753=CARTESIAN_POINT('Ctrl Pts',(0.842003832680442,-8.06424348185414,
5.52145719578458));
#31754=CARTESIAN_POINT('Ctrl Pts',(0.861753353595387,-8.87610181416697,
4.09068498337726));
#31755=CARTESIAN_POINT('Ctrl Pts',(0.881502874510331,-9.29832255855935,
2.55270144722397));
#31756=CARTESIAN_POINT('Ctrl Pts',(0.892163270394199,-9.52622886094455,
1.72252873423131));
#31757=CARTESIAN_POINT('Ctrl Pts',(0.902823666278068,-9.64060941270616,
0.861118670477449));
#31758=CARTESIAN_POINT('Ctrl Pts',(0.913484062161936,-9.64080718149228,
-0.000193112876372633));
#31759=CARTESIAN_POINT('Ctrl Pts',(-8.,-2.60344811511687,9.71940883564398));
#31760=CARTESIAN_POINT('Ctrl Pts',(-8.,-2.84069175470075,9.6506071796457));
#31761=CARTESIAN_POINT('Ctrl Pts',(-8.,-3.07490729689743,9.57303453428213));
#31762=CARTESIAN_POINT('Ctrl Pts',(-8.,-3.30569495421949,9.4870393850882));
#31763=CARTESIAN_POINT('Ctrl Pts',(-8.,-3.53907133521668,9.40007963630845));
#31764=CARTESIAN_POINT('Ctrl Pts',(-8.,-3.76894306703271,9.30450711868265));
#31765=CARTESIAN_POINT('Ctrl Pts',(-8.,-3.9948840188511,9.20063005080582));
#31766=CARTESIAN_POINT('Ctrl Pts',(-8.,-4.22183166262119,9.09629015311723));
#31767=CARTESIAN_POINT('Ctrl Pts',(-8.,-4.44481399609299,8.98357122395935));
#31768=CARTESIAN_POINT('Ctrl Pts',(-8.,-4.66337776867861,8.86273771780899));
#31769=CARTESIAN_POINT('Ctrl Pts',(-8.,-4.88031678224955,8.74280246357875));
#31770=CARTESIAN_POINT('Ctrl Pts',(-8.,-5.09290319963608,8.61487244542648));
#31771=CARTESIAN_POINT('Ctrl Pts',(-8.,-5.30066469035802,8.47916451832081));
#31772=CARTESIAN_POINT('Ctrl Pts',(-8.,-5.43935748628783,8.3885716381161));
#31773=CARTESIAN_POINT('Ctrl Pts',(-8.,-5.57589952659966,8.29451181350657));
#31774=CARTESIAN_POINT('Ctrl Pts',(-8.,-5.71014126262514,8.19704032519922));
#31775=CARTESIAN_POINT('Ctrl Pts',(-8.,-5.81242682170959,8.12277187507713));
#31776=CARTESIAN_POINT('Ctrl Pts',(-8.,-5.91337675491332,8.04652256746091));
#31777=CARTESIAN_POINT('Ctrl Pts',(-8.,-6.01292162257584,7.96831424157311));
#31778=CARTESIAN_POINT('Ctrl Pts',(-8.,-6.03974603533308,7.94723939900283));
#31779=CARTESIAN_POINT('Ctrl Pts',(-8.,-6.06647083477937,7.92602027127446));
#31780=CARTESIAN_POINT('Ctrl Pts',(-8.,-6.09307507746351,7.9046731501823));
#31781=CARTESIAN_POINT('Ctrl Pts',(-8.,-6.28715186618783,7.74894683392287));
#31782=CARTESIAN_POINT('Ctrl Pts',(-8.,-6.47502703975548,7.58624877613549));
#31783=CARTESIAN_POINT('Ctrl Pts',(-8.,-6.65627736318776,7.41686224654094));
#31784=CARTESIAN_POINT('Ctrl Pts',(-8.,-6.72100538512745,7.35637101653228));
#31785=CARTESIAN_POINT('Ctrl Pts',(-8.,-6.78488825702186,7.29502636554285));
#31786=CARTESIAN_POINT('Ctrl Pts',(-8.,-6.84790578274569,7.23283987189571));
#31787=CARTESIAN_POINT('Ctrl Pts',(-8.,-7.02385876529317,7.05920723707383));
#31788=CARTESIAN_POINT('Ctrl Pts',(-8.,-7.1930682957411,6.87901432974266));
#31789=CARTESIAN_POINT('Ctrl Pts',(-8.,-7.35530118613631,6.69274140140207));
#31790=CARTESIAN_POINT('Ctrl Pts',(-8.,-7.51824283162384,6.50565469303081));
#31791=CARTESIAN_POINT('Ctrl Pts',(-8.,-7.67414710687603,6.31243416749467));
#31792=CARTESIAN_POINT('Ctrl Pts',(-8.,-7.82273680022787,6.1135333512058));
#31793=CARTESIAN_POINT('Ctrl Pts',(-8.,-7.97083957648109,5.91528431773037));
#31794=CARTESIAN_POINT('Ctrl Pts',(-8.,-8.11167594519281,5.71139157758446));
#31795=CARTESIAN_POINT('Ctrl Pts',(-8.,-8.24492583126938,5.50228004576333));
#31796=CARTESIAN_POINT('Ctrl Pts',(-8.,-8.30521404253229,5.40766863123126));
#31797=CARTESIAN_POINT('Ctrl Pts',(-8.,-8.36394860502083,5.31198862209827));
#31798=CARTESIAN_POINT('Ctrl Pts',(-8.,-8.42109652453534,5.21527822770044));
#31799=CARTESIAN_POINT('Ctrl Pts',(-8.,-8.45087437095415,5.16488571479801));
#31800=CARTESIAN_POINT('Ctrl Pts',(-8.,-8.48022139245109,5.1142134322457));
#31801=CARTESIAN_POINT('Ctrl Pts',(-8.,-8.50913268358154,5.06326672997545));
#31802=CARTESIAN_POINT('Ctrl Pts',(-8.,-8.52853358179917,5.02907898717248));
#31803=CARTESIAN_POINT('Ctrl Pts',(-8.,-8.54774116172179,4.99476229317982));
#31804=CARTESIAN_POINT('Ctrl Pts',(-8.,-8.566737596633,4.96034817438508));
#31805=CARTESIAN_POINT('Ctrl Pts',(-8.,-8.68625360214662,4.74383186325392));
#31806=CARTESIAN_POINT('Ctrl Pts',(-8.,-8.79751972018929,4.52328352045298));
#31807=CARTESIAN_POINT('Ctrl Pts',(-8.,-8.90031166290089,4.29917501917082));
#31808=CARTESIAN_POINT('Ctrl Pts',(-8.,-9.00301013530597,4.07527030322198));
#31809=CARTESIAN_POINT('Ctrl Pts',(-8.,-9.09725014289365,3.8478113152238));
#31810=CARTESIAN_POINT('Ctrl Pts',(-8.,-9.18276362084067,3.61724207015639));
#31811=CARTESIAN_POINT('Ctrl Pts',(-8.,-9.25013085907205,3.43560037303228));
#31812=CARTESIAN_POINT('Ctrl Pts',(-8.,-9.3120813902539,3.2520277614531));
#31813=CARTESIAN_POINT('Ctrl Pts',(-8.,-9.36846282230467,3.06673324765561));
#31814=CARTESIAN_POINT('Ctrl Pts',(-8.,-9.44021345233254,2.83092869956063));
#31815=CARTESIAN_POINT('Ctrl Pts',(-8.,-9.50294661414108,2.59233538545246));
#31816=CARTESIAN_POINT('Ctrl Pts',(-8.,-9.55662994873875,2.35147811162457));
#31817=CARTESIAN_POINT('Ctrl Pts',(-8.,-9.59403316915113,2.18366369084712));
#31818=CARTESIAN_POINT('Ctrl Pts',(-8.,-9.62704213125647,2.01475001121834));
#31819=CARTESIAN_POINT('Ctrl Pts',(-8.,-9.65563094000264,1.84491408895825));
#31820=CARTESIAN_POINT('Ctrl Pts',(-8.,-9.66985498260186,1.76041412204629));
#31821=CARTESIAN_POINT('Ctrl Pts',(-8.,-9.68298464758163,1.67568586609032));
#31822=CARTESIAN_POINT('Ctrl Pts',(-8.,-9.6950156054378,1.59075123501256));
#31823=CARTESIAN_POINT('Ctrl Pts',(-8.,-9.70329987511925,1.53226699813347));
#31824=CARTESIAN_POINT('Ctrl Pts',(-8.,-9.71106318630873,1.47368491207996));
#31825=CARTESIAN_POINT('Ctrl Pts',(-8.,-9.71830391560107,1.41501216875315));
#31826=CARTESIAN_POINT('Ctrl Pts',(-8.,-9.72177711672372,1.38686828575954));
#31827=CARTESIAN_POINT('Ctrl Pts',(-8.,-9.7251301421797,1.35870260813857));
#31828=CARTESIAN_POINT('Ctrl Pts',(-8.,-9.72836100509793,1.33053262617027));
#31829=CARTESIAN_POINT('Ctrl Pts',(-8.,-9.75621794121566,1.08764723982277));
#31830=CARTESIAN_POINT('Ctrl Pts',(-8.,-9.77503407585364,0.844154007688625));
#31831=CARTESIAN_POINT('Ctrl Pts',(-8.,-9.78485423076769,0.600570555568447));
#31832=CARTESIAN_POINT('Ctrl Pts',(-8.,-9.7947445628712,0.35524639750051));
#31833=CARTESIAN_POINT('Ctrl Pts',(-8.,-9.79550994101194,0.109830070692749));
#31834=CARTESIAN_POINT('Ctrl Pts',(-8.,-9.78714425198491,-0.135157548107968));
#31835=CARTESIAN_POINT('Ctrl Pts',(-8.,-9.77880540331052,-0.379359152264971));
#31836=CARTESIAN_POINT('Ctrl Pts',(-8.,-9.76139396821941,-0.623135449836081));
#31837=CARTESIAN_POINT('Ctrl Pts',(-8.,-9.73485231894389,-0.865968566157455));
#31838=CARTESIAN_POINT('Ctrl Pts',(-8.,-9.70865278207418,-1.10567165009949));
#31839=CARTESIAN_POINT('Ctrl Pts',(-8.,-9.67355679806456,-1.34445630895454));
#31840=CARTESIAN_POINT('Ctrl Pts',(-8.,-9.62945950106302,-1.58181321655475));
#31841=CARTESIAN_POINT('Ctrl Pts',(-8.,-9.61925297631356,-1.63675057817564));
#31842=CARTESIAN_POINT('Ctrl Pts',(-8.,-9.60856403154122,-1.69161138395428));
#31843=CARTESIAN_POINT('Ctrl Pts',(-8.,-9.59739098933044,-1.74638917930737));
#31844=CARTESIAN_POINT('Ctrl Pts',(-8.,-9.55734323407315,-1.94273031008005));
#31845=CARTESIAN_POINT('Ctrl Pts',(-8.,-9.51107764561208,-2.13800587130263));
#31846=CARTESIAN_POINT('Ctrl Pts',(-8.,-9.45868909970552,-2.33194442065493));
#31847=CARTESIAN_POINT('Ctrl Pts',(-8.,-9.44806059824241,-2.37129035247791));
#31848=CARTESIAN_POINT('Ctrl Pts',(-8.,-9.43717863430331,-2.41058583297454));
#31849=CARTESIAN_POINT('Ctrl Pts',(-8.,-9.42605224583319,-2.44979983523773));
#31850=CARTESIAN_POINT('Ctrl Pts',(-8.,-9.35956117403027,-2.68414191732166));
#31851=CARTESIAN_POINT('Ctrl Pts',(-8.,-9.28429949582149,-2.91575310001084));
#31852=CARTESIAN_POINT('Ctrl Pts',(-8.,-9.20053845138115,-3.14417928716639));
#31853=CARTESIAN_POINT('Ctrl Pts',(-8.,-9.11644481764174,-3.37351248432862));
#31854=CARTESIAN_POINT('Ctrl Pts',(-8.,-9.02378391065593,-3.59963594961518));
#31855=CARTESIAN_POINT('Ctrl Pts',(-8.,-8.92278109081723,-3.82207193311861));
#31856=CARTESIAN_POINT('Ctrl Pts',(-8.,-8.83217822033651,-4.02160436831));
#31857=CARTESIAN_POINT('Ctrl Pts',(-8.,-8.73486208468608,-4.21816966332805));
#31858=CARTESIAN_POINT('Ctrl Pts',(-8.,-8.63096467988468,-4.41140451002018));
#31859=CARTESIAN_POINT('Ctrl Pts',(-8.,-8.6132277370607,-4.44439277795555));
#31860=CARTESIAN_POINT('Ctrl Pts',(-8.,-8.59529892556715,-4.47728393468828));
#31861=CARTESIAN_POINT('Ctrl Pts',(-8.,-8.57717882354457,-4.51007610976465));
#31862=CARTESIAN_POINT('Ctrl Pts',(-8.,-8.56101088203111,-4.5393354355716));
#31863=CARTESIAN_POINT('Ctrl Pts',(-8.,-8.54469193487426,-4.56851355146286));
#31864=CARTESIAN_POINT('Ctrl Pts',(-8.,-8.52822778415311,-4.59759995652038));
#31865=CARTESIAN_POINT('Ctrl Pts',(-8.,-8.40828066692113,-4.80950462724276));
#31866=CARTESIAN_POINT('Ctrl Pts',(-8.,-8.28055244077711,-5.01668533600614));
#31867=CARTESIAN_POINT('Ctrl Pts',(-8.,-8.14527403028023,-5.21867499254995));
#31868=CARTESIAN_POINT('Ctrl Pts',(-8.,-8.01107409605472,-5.41905433262977));
#31869=CARTESIAN_POINT('Ctrl Pts',(-8.,-7.86944352784287,-5.61432559405275));
#31870=CARTESIAN_POINT('Ctrl Pts',(-8.,-7.72056574116336,-5.80400386624563));
#31871=CARTESIAN_POINT('Ctrl Pts',(-8.,-7.65750042133828,-5.8843524606633));
#31872=CARTESIAN_POINT('Ctrl Pts',(-8.,-7.59313416638248,-5.96369704112626));
#31873=CARTESIAN_POINT('Ctrl Pts',(-8.,-7.52747884839902,-6.0419988087639));
#31874=CARTESIAN_POINT('Ctrl Pts',(-8.,-7.42746572080017,-6.1612763466464));
#31875=CARTESIAN_POINT('Ctrl Pts',(-8.,-7.32446159078778,-6.27813441156677));
#31876=CARTESIAN_POINT('Ctrl Pts',(-8.,-7.21857424983126,-6.39248700007983));
#31877=CARTESIAN_POINT('Origin',(-8.,12.5,0.));
#31878=CARTESIAN_POINT('',(-8.,-12.5,-1.53080849893419E-15));
#31879=CARTESIAN_POINT('Origin',(-8.,0.,0.));
#31880=CARTESIAN_POINT('Origin',(-3.5,0.,0.));
#31881=CARTESIAN_POINT('Origin',(-4.,0.,0.));
#31882=CARTESIAN_POINT('',(0.,-12.5,-1.53080849893419E-15));
#31883=CARTESIAN_POINT('Origin',(0.,0.,0.));
#31884=CARTESIAN_POINT('',(-4.,-12.5,-1.53080849893419E-15));
#31885=CARTESIAN_POINT('Origin',(0.,13.5,0.));
#31886=CARTESIAN_POINT('',(0.,-13.5,-1.65327317884893E-15));
#31887=CARTESIAN_POINT('Origin',(0.,0.,0.));
#31888=CARTESIAN_POINT('Origin',(0.3,0.,0.));
#31889=CARTESIAN_POINT('',(0.6,-13.5,-1.65327317884893E-15));
#31890=CARTESIAN_POINT('Origin',(0.6,0.,0.));
#31891=CARTESIAN_POINT('',(0.3,-13.5,-1.65327317884893E-15));
#31892=CARTESIAN_POINT('Origin',(0.8,0.,0.));
#31893=CARTESIAN_POINT('',(1.,-13.1,-1.60428730688303E-15));
#31894=CARTESIAN_POINT('Origin',(1.,0.,0.));
#31895=CARTESIAN_POINT('',(0.8,-13.3,-1.62878024286598E-15));
#31896=CARTESIAN_POINT('Origin',(1.,9.6,0.));
#38504=UNCERTAINTY_MEASURE_WITH_UNIT(LENGTH_MEASURE(0.01),#38529,
'DISTANCE_ACCURACY_VALUE',
'Maximum model space distance between geometric entities at asserted c
onnectivities');
#38514=UNCERTAINTY_MEASURE_WITH_UNIT(LENGTH_MEASURE(0.01),#38529,
'DISTANCE_ACCURACY_VALUE',
'Maximum model space distance between geometric entities at asserted c
onnectivities');
#38518=(
GEOMETRIC_REPRESENTATION_CONTEXT(3)
GLOBAL_UNCERTAINTY_ASSIGNED_CONTEXT((#38504))
GLOBAL_UNIT_ASSIGNED_CONTEXT((#38529,#38531,#38532))
REPRESENTATION_CONTEXT('','3D')
);
#38528=(
GEOMETRIC_REPRESENTATION_CONTEXT(3)
GLOBAL_UNCERTAINTY_ASSIGNED_CONTEXT((#38514))
GLOBAL_UNIT_ASSIGNED_CONTEXT((#38529,#38531,#38532))
REPRESENTATION_CONTEXT('','3D')
);
#38529=(
LENGTH_UNIT()
NAMED_UNIT(*)
SI_UNIT(.MILLI.,.METRE.)
);
#38531=(
NAMED_UNIT(*)
PLANE_ANGLE_UNIT()
SI_UNIT($,.RADIAN.)
);
#38532=(
NAMED_UNIT(*)
SI_UNIT($,.STERADIAN.)
SOLID_ANGLE_UNIT()
);
#38536=SHAPE_DEFINITION_REPRESENTATION(#38549,#38578);
#38549=PRODUCT_DEFINITION_SHAPE('',$,#38592);
#38578=SHAPE_REPRESENTATION('',(#18599),#38518);
#38588=PRODUCT_DEFINITION_CONTEXT('part definition',#38629,'design');
#38592=PRODUCT_DEFINITION('2026-10-20-13-39-07-742',
'03_Brass_RMS_Objective_Socket',#38605,#38588);
#38605=PRODUCT_DEFINITION_FORMATION('',$,#38634);
#38629=APPLICATION_CONTEXT(
'Core Data for Automotive Mechanical Design Process');
#38630=PRODUCT_CONTEXT('part definition',#38629,'mechanical');
#38634=PRODUCT('2026-10-20-13-39-07-742',
'03_Brass_RMS_Objective_Socket',$,(#38630));
#38686=COLOUR_RGB('Light Blue',0.38,0.62,0.78);
#38687=FILL_AREA_STYLE_COLOUR('',#38686);
#38688=FILL_AREA_STYLE('',(#38687));
#38689=SURFACE_STYLE_FILL_AREA(#38688);
#38690=SURFACE_SIDE_STYLE('',(#38689));
#38691=SURFACE_STYLE_USAGE(.BOTH.,#38690);
#38692=PRESENTATION_STYLE_ASSIGNMENT((#38691));
ENDSEC;
END-ISO-10303-21;
